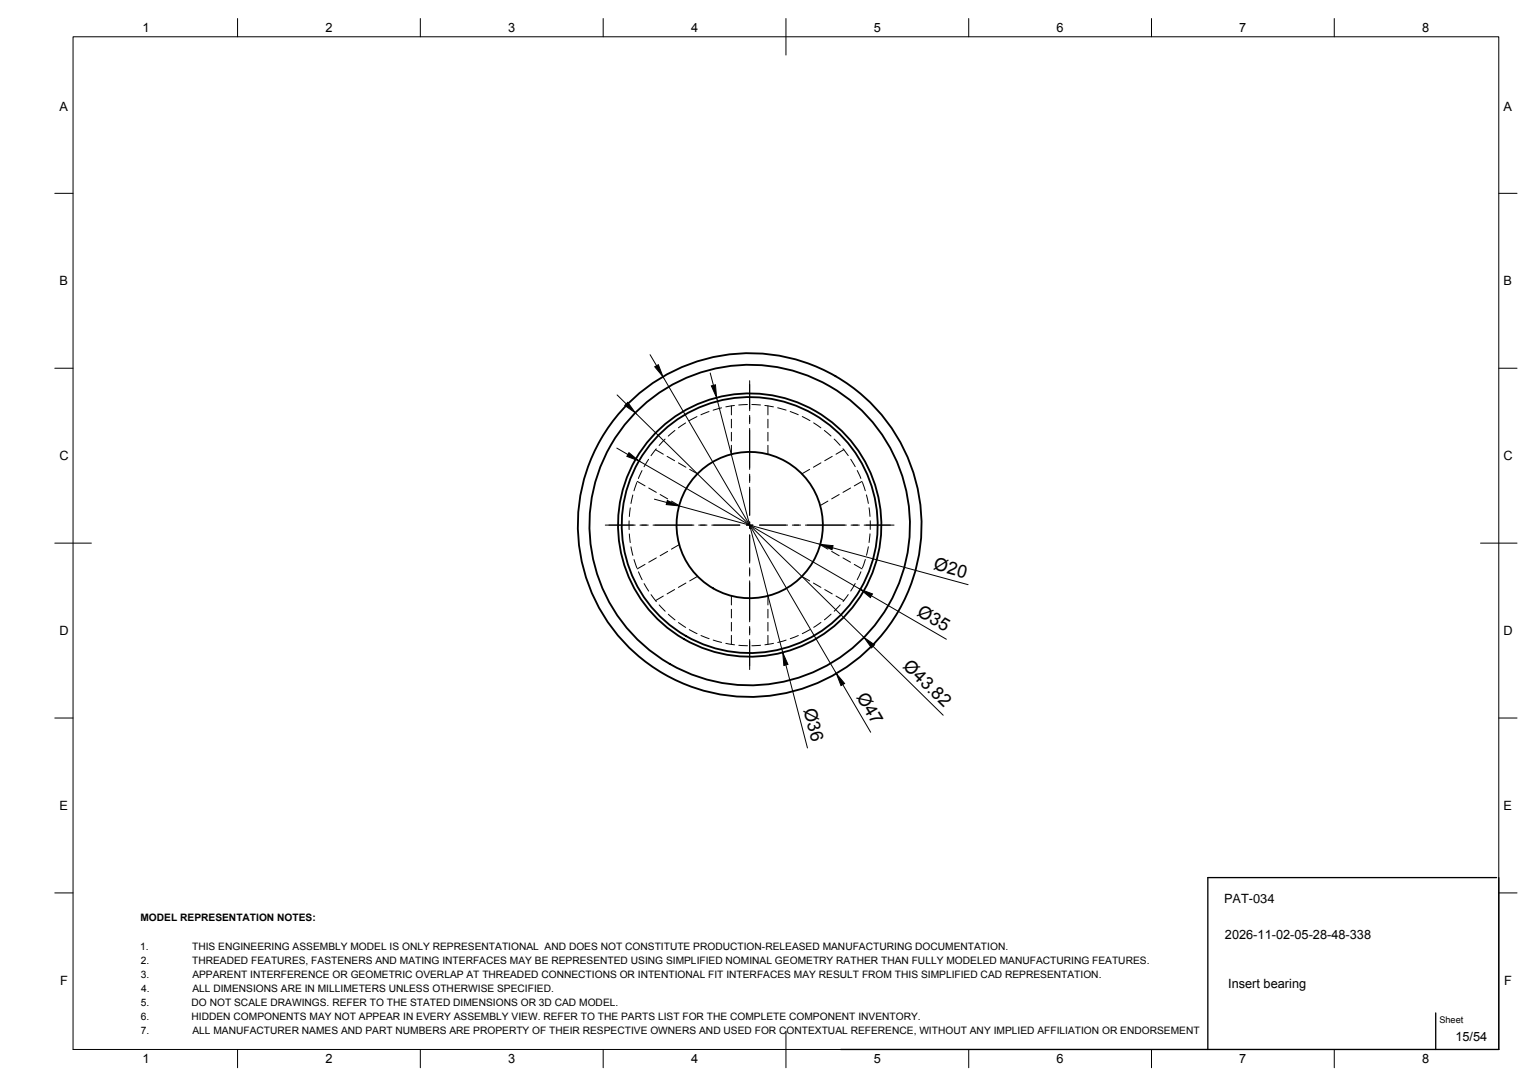
ISO-10303-21;
HEADER;
/* Generated by software containing ST-Developer
 * from STEP Tools, Inc. (www.steptools.com) 
 */

FILE_DESCRIPTION(
/* description */ ('Fatigue rig crank-slider'),
/* implementation_level */ '2;1');

FILE_NAME(
/* name */ 'Insert bearing.step',
/* time_stamp */ '2026-10-28T03:24:50-07:00',
/* author */ (''),
/* organization */ (''),
/* preprocessor_version */ 'ST-DEVELOPER v20.2',
/* originating_system */ 'Autodesk Translation Framework v15.17.0.0',
/* authorisation */ '');

FILE_SCHEMA (('AUTOMOTIVE_DESIGN { 1 0 10303 214 3 1 1 }'));
ENDSEC;

DATA;
#10=MECHANICAL_DESIGN_GEOMETRIC_PRESENTATION_REPRESENTATION('',(#598,#599),#16911);
#415=B_SPLINE_CURVE_WITH_KNOTS('',3,(#14016,#14017,#14018,#14019,#14020,
#14021,#14022,#14023,#14024,#14025),.UNSPECIFIED.,.F.,.F.,(4,2,2,2,4),(1.13193471301885,
1.22626174930539,1.32058878559194,1.41491753480854,1.50924628402513),
 .UNSPECIFIED.);
#416=B_SPLINE_CURVE_WITH_KNOTS('',3,(#14027,#14028,#14029,#14030,#14031,
#14032,#14033,#14034,#14035,#14036,#14037,#14038,#14039,#14040,#14041,#14042,
#14043,#14044),.UNSPECIFIED.,.F.,.F.,(4,2,2,2,2,2,2,2,4),(0.377311571006283,
0.471638607292829,0.565965643579376,0.66029439279597,0.754623142012565,
0.84895189122916,0.943280640445754,1.0376076767323,1.13193471301885),
 .UNSPECIFIED.);
#417=B_SPLINE_CURVE_WITH_KNOTS('',3,(#14045,#14046,#14047,#14048,#14049,
#14050,#14051,#14052,#14053,#14054),.UNSPECIFIED.,.F.,.F.,(4,2,2,2,4),(1.50924628402513,
1.60357503324173,1.69790378245832,1.79223081874487,1.88655785503141),
 .UNSPECIFIED.);
#418=B_SPLINE_CURVE_WITH_KNOTS('',3,(#14057,#14058,#14059,#14060,#14061,
#14062,#14063,#14064,#14065,#14066,#14067,#14068,#14069,#14070,#14071,#14072,
#14073,#14074,#14075,#14076,#14077,#14078,#14079,#14080,#14081,#14082,#14083,
#14084,#14085,#14086,#14087,#14088,#14089,#14090),.UNSPECIFIED.,.T.,.F.,
(4,2,2,2,2,2,2,2,2,2,2,2,2,2,2,2,4),(0.,0.0946120580087934,0.189224116017587,
0.283822945575014,0.378421775132442,0.47302060468987,0.567619434247297,
0.662231492256091,0.756843550264884,0.851455608273677,0.94606766628247,
1.0406664958399,1.13526532539733,1.22986415495475,1.32446298451218,1.41907504252097,
1.51368710052977),.UNSPECIFIED.);
#419=B_SPLINE_CURVE_WITH_KNOTS('',3,(#14093,#14094,#14095,#14096,#14097,
#14098,#14099,#14100,#14101,#14102,#14103,#14104,#14105,#14106,#14107,#14108,
#14109,#14110,#14111,#14112,#14113,#14114,#14115,#14116,#14117,#14118,#14119,
#14120,#14121,#14122,#14123,#14124,#14125,#14126),.UNSPECIFIED.,.T.,.F.,
(4,2,2,2,2,2,2,2,2,2,2,2,2,2,2,2,4),(0.,0.0946120580087934,0.189224116017587,
0.283822945575014,0.378421775132442,0.47302060468987,0.567619434247297,
0.66223149225609,0.756843550264884,0.851455608273677,0.94606766628247,1.0406664958399,
1.13526532539733,1.22986415495475,1.32446298451218,1.41907504252097,1.51368710052977),
 .UNSPECIFIED.);
#420=B_SPLINE_CURVE_WITH_KNOTS('',3,(#14130,#14131,#14132,#14133,#14134,
#14135,#14136,#14137,#14138,#14139),.UNSPECIFIED.,.F.,.F.,(4,2,2,2,4),(1.13193471301885,
1.22626174930539,1.32058878559194,1.41491753480854,1.50924628402513),
 .UNSPECIFIED.);
#421=B_SPLINE_CURVE_WITH_KNOTS('',3,(#14141,#14142,#14143,#14144,#14145,
#14146,#14147,#14148,#14149,#14150,#14151,#14152,#14153,#14154,#14155,#14156,
#14157,#14158),.UNSPECIFIED.,.F.,.F.,(4,2,2,2,2,2,2,2,4),(0.377311571006283,
0.47163860729283,0.565965643579376,0.660294392795971,0.754623142012565,
0.84895189122916,0.943280640445755,1.0376076767323,1.13193471301885),
 .UNSPECIFIED.);
#422=B_SPLINE_CURVE_WITH_KNOTS('',3,(#14159,#14160,#14161,#14162,#14163,
#14164,#14165,#14166,#14167,#14168),.UNSPECIFIED.,.F.,.F.,(4,2,2,2,4),(1.50924628402513,
1.60357503324173,1.69790378245832,1.79223081874487,1.88655785503141),
 .UNSPECIFIED.);
#423=B_SPLINE_CURVE_WITH_KNOTS('',3,(#14177,#14178,#14179,#14180,#14181,
#14182,#14183,#14184,#14185,#14186,#14187,#14188,#14189,#14190,#14191,#14192,
#14193,#14194),.UNSPECIFIED.,.F.,.F.,(4,2,2,2,2,2,2,2,4),(0.377311571006282,
0.471638607292829,0.565965643579376,0.660294392795971,0.754623142012565,
0.84895189122916,0.943280640445754,1.0376076767323,1.13193471301885),
 .UNSPECIFIED.);
#424=B_SPLINE_CURVE_WITH_KNOTS('',3,(#14196,#14197,#14198,#14199,#14200,
#14201,#14202,#14203,#14204,#14205),.UNSPECIFIED.,.F.,.F.,(4,2,2,2,4),(1.13193471301885,
1.22626174930539,1.32058878559194,1.41491753480854,1.50924628402513),
 .UNSPECIFIED.);
#425=B_SPLINE_CURVE_WITH_KNOTS('',3,(#14206,#14207,#14208,#14209,#14210,
#14211,#14212,#14213,#14214,#14215),.UNSPECIFIED.,.F.,.F.,(4,2,2,2,4),(1.50924628402513,
1.60357503324172,1.69790378245832,1.79223081874487,1.88655785503141),
 .UNSPECIFIED.);
#426=B_SPLINE_CURVE_WITH_KNOTS('',3,(#14218,#14219,#14220,#14221,#14222,
#14223,#14224,#14225,#14226,#14227,#14228,#14229,#14230,#14231,#14232,#14233,
#14234,#14235),.UNSPECIFIED.,.F.,.F.,(4,2,2,2,2,2,2,2,4),(0.377311571006283,
0.47163860729283,0.565965643579376,0.660294392795971,0.754623142012565,
0.84895189122916,0.943280640445754,1.0376076767323,1.13193471301885),
 .UNSPECIFIED.);
#427=B_SPLINE_CURVE_WITH_KNOTS('',3,(#14237,#14238,#14239,#14240,#14241,
#14242,#14243,#14244,#14245,#14246),.UNSPECIFIED.,.F.,.F.,(4,2,2,2,4),(1.13193471301885,
1.22626174930539,1.32058878559194,1.41491753480854,1.50924628402513),
 .UNSPECIFIED.);
#428=B_SPLINE_CURVE_WITH_KNOTS('',3,(#14247,#14248,#14249,#14250,#14251,
#14252,#14253,#14254,#14255,#14256),.UNSPECIFIED.,.F.,.F.,(4,2,2,2,4),(1.50924628402513,
1.60357503324173,1.69790378245832,1.79223081874487,1.88655785503141),
 .UNSPECIFIED.);
#429=B_SPLINE_CURVE_WITH_KNOTS('',3,(#14259,#14260,#14261,#14262,#14263,
#14264,#14265,#14266,#14267,#14268,#14269,#14270,#14271,#14272,#14273,#14274,
#14275,#14276),.UNSPECIFIED.,.F.,.F.,(4,2,2,2,2,2,2,2,4),(0.377311571006282,
0.471638607292829,0.565965643579376,0.66029439279597,0.754623142012565,
0.84895189122916,0.943280640445754,1.0376076767323,1.13193471301885),
 .UNSPECIFIED.);
#430=B_SPLINE_CURVE_WITH_KNOTS('',3,(#14278,#14279,#14280,#14281,#14282,
#14283,#14284,#14285,#14286,#14287),.UNSPECIFIED.,.F.,.F.,(4,2,2,2,4),(1.13193471301885,
1.22626174930539,1.32058878559194,1.41491753480854,1.50924628402513),
 .UNSPECIFIED.);
#431=B_SPLINE_CURVE_WITH_KNOTS('',3,(#14288,#14289,#14290,#14291,#14292,
#14293,#14294,#14295,#14296,#14297),.UNSPECIFIED.,.F.,.F.,(4,2,2,2,4),(1.50924628402513,
1.60357503324172,1.69790378245832,1.79223081874487,1.88655785503141),
 .UNSPECIFIED.);
#432=B_SPLINE_CURVE_WITH_KNOTS('',3,(#14300,#14301,#14302,#14303,#14304,
#14305,#14306,#14307,#14308,#14309,#14310,#14311,#14312,#14313,#14314,#14315,
#14316,#14317),.UNSPECIFIED.,.F.,.F.,(4,2,2,2,2,2,2,2,4),(0.377311571006283,
0.471638607292829,0.565965643579376,0.660294392795971,0.754623142012565,
0.84895189122916,0.943280640445755,1.0376076767323,1.13193471301885),
 .UNSPECIFIED.);
#433=B_SPLINE_CURVE_WITH_KNOTS('',3,(#14319,#14320,#14321,#14322,#14323,
#14324,#14325,#14326,#14327,#14328),.UNSPECIFIED.,.F.,.F.,(4,2,2,2,4),(1.13193471301885,
1.22626174930539,1.32058878559194,1.41491753480854,1.50924628402513),
 .UNSPECIFIED.);
#434=B_SPLINE_CURVE_WITH_KNOTS('',3,(#14329,#14330,#14331,#14332,#14333,
#14334,#14335,#14336,#14337,#14338),.UNSPECIFIED.,.F.,.F.,(4,2,2,2,4),(1.50924628402513,
1.60357503324172,1.69790378245832,1.79223081874487,1.88655785503141),
 .UNSPECIFIED.);
#435=B_SPLINE_CURVE_WITH_KNOTS('',3,(#14342,#14343,#14344,#14345,#14346,
#14347,#14348,#14349,#14350,#14351,#14352,#14353,#14354,#14355,#14356,#14357,
#14358,#14359,#14360,#14361,#14362,#14363,#14364,#14365,#14366,#14367,#14368,
#14369,#14370,#14371,#14372,#14373,#14374,#14375),.UNSPECIFIED.,.T.,.F.,
(4,2,2,2,2,2,2,2,2,2,2,2,2,2,2,2,4),(0.,0.0946120580087934,0.189224116017587,
0.283822945575014,0.378421775132442,0.47302060468987,0.567619434247297,
0.66223149225609,0.756843550264884,0.851455608273677,0.94606766628247,1.0406664958399,
1.13526532539733,1.22986415495475,1.32446298451218,1.41907504252097,1.51368710052977),
 .UNSPECIFIED.);
#436=B_SPLINE_CURVE_WITH_KNOTS('',3,(#14378,#14379,#14380,#14381,#14382,
#14383,#14384,#14385,#14386,#14387,#14388,#14389,#14390,#14391,#14392,#14393,
#14394,#14395,#14396,#14397,#14398,#14399,#14400,#14401,#14402,#14403,#14404,
#14405,#14406,#14407,#14408,#14409,#14410,#14411),.UNSPECIFIED.,.T.,.F.,
(4,2,2,2,2,2,2,2,2,2,2,2,2,2,2,2,4),(0.,0.0946120580087934,0.189224116017587,
0.283822945575014,0.378421775132442,0.47302060468987,0.567619434247297,
0.66223149225609,0.756843550264884,0.851455608273677,0.94606766628247,1.0406664958399,
1.13526532539733,1.22986415495475,1.32446298451218,1.41907504252097,1.51368710052977),
 .UNSPECIFIED.);
#437=B_SPLINE_CURVE_WITH_KNOTS('',3,(#14416,#14417,#14418,#14419,#14420,
#14421,#14422,#14423,#14424,#14425,#14426,#14427,#14428,#14429,#14430,#14431,
#14432,#14433,#14434,#14435,#14436,#14437,#14438,#14439,#14440,#14441,#14442,
#14443,#14444,#14445,#14446,#14447,#14448,#14449),.UNSPECIFIED.,.T.,.F.,
(4,2,2,2,2,2,2,2,2,2,2,2,2,2,2,2,4),(0.,0.0946120580087934,0.189224116017587,
0.283822945575014,0.378421775132442,0.47302060468987,0.567619434247297,
0.66223149225609,0.756843550264884,0.851455608273677,0.94606766628247,1.0406664958399,
1.13526532539733,1.22986415495475,1.32446298451218,1.41907504252097,1.51368710052977),
 .UNSPECIFIED.);
#438=B_SPLINE_CURVE_WITH_KNOTS('',3,(#14452,#14453,#14454,#14455,#14456,
#14457,#14458,#14459,#14460,#14461,#14462,#14463,#14464,#14465,#14466,#14467,
#14468,#14469,#14470,#14471,#14472,#14473,#14474,#14475,#14476,#14477,#14478,
#14479,#14480,#14481,#14482,#14483,#14484,#14485),.UNSPECIFIED.,.T.,.F.,
(4,2,2,2,2,2,2,2,2,2,2,2,2,2,2,2,4),(0.,0.0946120580087934,0.189224116017587,
0.283822945575014,0.378421775132442,0.47302060468987,0.567619434247297,
0.66223149225609,0.756843550264884,0.851455608273677,0.94606766628247,1.0406664958399,
1.13526532539733,1.22986415495475,1.32446298451218,1.41907504252097,1.51368710052977),
 .UNSPECIFIED.);
#470=SPHERICAL_SURFACE('',#9773,2.35);
#498=SHAPE_REPRESENTATION_RELATIONSHIP('SRR','None',#17138,#548);
#548=ADVANCED_BREP_SHAPE_REPRESENTATION('',(#657,#658),#16867);
#598=STYLED_ITEM('',(#17487),#657);
#599=STYLED_ITEM('',(#17487),#658);
#657=MANIFOLD_SOLID_BREP('Body1',#8889);
#658=MANIFOLD_SOLID_BREP('Body2',#8890);
#786=FACE_BOUND('',#1969,.T.);
#787=FACE_BOUND('',#1971,.T.);
#788=FACE_BOUND('',#1972,.T.);
#789=FACE_BOUND('',#1974,.T.);
#790=FACE_BOUND('',#1978,.T.);
#791=FACE_BOUND('',#1979,.T.);
#792=FACE_BOUND('',#1980,.T.);
#793=FACE_BOUND('',#1981,.T.);
#794=FACE_BOUND('',#1982,.T.);
#795=FACE_BOUND('',#1983,.T.);
#796=FACE_BOUND('',#1989,.T.);
#797=FACE_BOUND('',#1991,.T.);
#798=FACE_BOUND('',#1994,.T.);
#799=FACE_BOUND('',#1996,.T.);
#800=FACE_BOUND('',#1997,.T.);
#801=FACE_BOUND('',#1998,.T.);
#802=FACE_BOUND('',#1999,.T.);
#803=FACE_BOUND('',#2000,.T.);
#804=FACE_BOUND('',#2001,.T.);
#980=PLANE('',#9771);
#981=PLANE('',#9776);
#982=PLANE('',#9786);
#983=PLANE('',#9788);
#984=PLANE('',#9792);
#1358=FACE_OUTER_BOUND('',#1967,.T.);
#1359=FACE_OUTER_BOUND('',#1968,.T.);
#1360=FACE_OUTER_BOUND('',#1970,.T.);
#1361=FACE_OUTER_BOUND('',#1973,.T.);
#1362=FACE_OUTER_BOUND('',#1975,.T.);
#1363=FACE_OUTER_BOUND('',#1976,.T.);
#1364=FACE_OUTER_BOUND('',#1977,.T.);
#1365=FACE_OUTER_BOUND('',#1984,.T.);
#1366=FACE_OUTER_BOUND('',#1985,.T.);
#1367=FACE_OUTER_BOUND('',#1986,.T.);
#1368=FACE_OUTER_BOUND('',#1987,.T.);
#1369=FACE_OUTER_BOUND('',#1988,.T.);
#1370=FACE_OUTER_BOUND('',#1990,.T.);
#1371=FACE_OUTER_BOUND('',#1992,.T.);
#1372=FACE_OUTER_BOUND('',#1993,.T.);
#1373=FACE_OUTER_BOUND('',#1995,.T.);
#1967=EDGE_LOOP('',(#6574,#6575,#6576,#6577));
#1968=EDGE_LOOP('',(#6578));
#1969=EDGE_LOOP('',(#6579));
#1970=EDGE_LOOP('',(#6580,#6581));
#1971=EDGE_LOOP('',(#6582));
#1972=EDGE_LOOP('',(#6583));
#1973=EDGE_LOOP('',(#6584));
#1974=EDGE_LOOP('',(#6585));
#1975=EDGE_LOOP('',(#6586,#6587,#6588,#6589,#6590,#6591));
#1976=EDGE_LOOP('',(#6592,#6593,#6594,#6595,#6596,#6597));
#1977=EDGE_LOOP('',(#6598,#6599,#6600,#6601));
#1978=EDGE_LOOP('',(#6602,#6603,#6604));
#1979=EDGE_LOOP('',(#6605,#6606,#6607));
#1980=EDGE_LOOP('',(#6608,#6609,#6610));
#1981=EDGE_LOOP('',(#6611,#6612,#6613));
#1982=EDGE_LOOP('',(#6614,#6615,#6616));
#1983=EDGE_LOOP('',(#6617,#6618,#6619));
#1984=EDGE_LOOP('',(#6620,#6621,#6622,#6623,#6624,#6625));
#1985=EDGE_LOOP('',(#6626,#6627,#6628,#6629,#6630,#6631));
#1986=EDGE_LOOP('',(#6632,#6633,#6634,#6635,#6636,#6637));
#1987=EDGE_LOOP('',(#6638,#6639,#6640,#6641,#6642,#6643));
#1988=EDGE_LOOP('',(#6644));
#1989=EDGE_LOOP('',(#6645));
#1990=EDGE_LOOP('',(#6646));
#1991=EDGE_LOOP('',(#6647));
#1992=EDGE_LOOP('',(#6648,#6649,#6650,#6651));
#1993=EDGE_LOOP('',(#6652));
#1994=EDGE_LOOP('',(#6653));
#1995=EDGE_LOOP('',(#6654,#6655,#6656,#6657));
#1996=EDGE_LOOP('',(#6658));
#1997=EDGE_LOOP('',(#6659));
#1998=EDGE_LOOP('',(#6660));
#1999=EDGE_LOOP('',(#6661));
#2000=EDGE_LOOP('',(#6662));
#2001=EDGE_LOOP('',(#6663));
#2630=LINE('',#14001,#3276);
#2631=LINE('',#14056,#3277);
#2632=LINE('',#14128,#3278);
#2633=LINE('',#14173,#3279);
#2634=LINE('',#14341,#3280);
#2635=LINE('',#14412,#3281);
#2636=LINE('',#14415,#3282);
#2637=LINE('',#14486,#3283);
#2638=LINE('',#14496,#3284);
#2639=LINE('',#14501,#3285);
#3276=VECTOR('',#11290,1.8);
#3277=VECTOR('',#11307,0.25);
#3278=VECTOR('',#11310,0.25);
#3279=VECTOR('',#11315,1.65);
#3280=VECTOR('',#11320,0.25);
#3281=VECTOR('',#11323,0.25);
#3282=VECTOR('',#11326,0.25);
#3283=VECTOR('',#11329,0.25);
#3284=VECTOR('',#11342,1.75);
#3285=VECTOR('',#11349,1.);
#3871=CIRCLE('',#9769,1.8);
#3872=CIRCLE('',#9770,1.8);
#3873=CIRCLE('',#9772,2.19089023002066);
#3874=CIRCLE('',#9774,2.35);
#3875=CIRCLE('',#9775,2.19089023002066);
#3876=CIRCLE('',#9780,1.65);
#3877=CIRCLE('',#9781,1.65);
#3878=CIRCLE('',#9787,1.);
#3879=CIRCLE('',#9789,1.75);
#3880=CIRCLE('',#9791,1.75);
#3881=CIRCLE('',#9793,1.);
#4346=VERTEX_POINT('',#13998);
#4347=VERTEX_POINT('',#14000);
#4348=VERTEX_POINT('',#14004);
#4349=VERTEX_POINT('',#14007);
#4350=VERTEX_POINT('',#14008);
#4351=VERTEX_POINT('',#14010);
#4352=VERTEX_POINT('',#14014);
#4353=VERTEX_POINT('',#14015);
#4354=VERTEX_POINT('',#14026);
#4355=VERTEX_POINT('',#14055);
#4356=VERTEX_POINT('',#14092);
#4357=VERTEX_POINT('',#14127);
#4358=VERTEX_POINT('',#14129);
#4359=VERTEX_POINT('',#14140);
#4360=VERTEX_POINT('',#14170);
#4361=VERTEX_POINT('',#14172);
#4362=VERTEX_POINT('',#14175);
#4363=VERTEX_POINT('',#14176);
#4364=VERTEX_POINT('',#14195);
#4365=VERTEX_POINT('',#14216);
#4366=VERTEX_POINT('',#14217);
#4367=VERTEX_POINT('',#14236);
#4368=VERTEX_POINT('',#14257);
#4369=VERTEX_POINT('',#14258);
#4370=VERTEX_POINT('',#14277);
#4371=VERTEX_POINT('',#14298);
#4372=VERTEX_POINT('',#14299);
#4373=VERTEX_POINT('',#14318);
#4374=VERTEX_POINT('',#14340);
#4375=VERTEX_POINT('',#14377);
#4376=VERTEX_POINT('',#14414);
#4377=VERTEX_POINT('',#14451);
#4378=VERTEX_POINT('',#14488);
#4379=VERTEX_POINT('',#14491);
#4380=VERTEX_POINT('',#14494);
#4381=VERTEX_POINT('',#14498);
#5185=EDGE_CURVE('',#4346,#4346,#3871,.T.);
#5186=EDGE_CURVE('',#4346,#4347,#2630,.T.);
#5187=EDGE_CURVE('',#4347,#4347,#3872,.T.);
#5188=EDGE_CURVE('',#4348,#4348,#3873,.T.);
#5189=EDGE_CURVE('',#4349,#4350,#3874,.T.);
#5190=EDGE_CURVE('',#4351,#4351,#3875,.T.);
#5191=EDGE_CURVE('',#4352,#4353,#415,.T.);
#5192=EDGE_CURVE('',#4354,#4352,#416,.T.);
#5193=EDGE_CURVE('',#4353,#4354,#417,.T.);
#5194=EDGE_CURVE('',#4353,#4355,#2631,.T.);
#5195=EDGE_CURVE('',#4355,#4355,#418,.T.);
#5196=EDGE_CURVE('',#4356,#4356,#419,.T.);
#5197=EDGE_CURVE('',#4356,#4357,#2632,.T.);
#5198=EDGE_CURVE('',#4358,#4357,#420,.T.);
#5199=EDGE_CURVE('',#4359,#4358,#421,.T.);
#5200=EDGE_CURVE('',#4357,#4359,#422,.T.);
#5201=EDGE_CURVE('',#4360,#4360,#3876,.T.);
#5202=EDGE_CURVE('',#4360,#4361,#2633,.T.);
#5203=EDGE_CURVE('',#4361,#4361,#3877,.T.);
#5204=EDGE_CURVE('',#4362,#4363,#423,.T.);
#5205=EDGE_CURVE('',#4363,#4364,#424,.T.);
#5206=EDGE_CURVE('',#4364,#4362,#425,.T.);
#5207=EDGE_CURVE('',#4365,#4366,#426,.T.);
#5208=EDGE_CURVE('',#4366,#4367,#427,.T.);
#5209=EDGE_CURVE('',#4367,#4365,#428,.T.);
#5210=EDGE_CURVE('',#4368,#4369,#429,.T.);
#5211=EDGE_CURVE('',#4369,#4370,#430,.T.);
#5212=EDGE_CURVE('',#4370,#4368,#431,.T.);
#5213=EDGE_CURVE('',#4371,#4372,#432,.T.);
#5214=EDGE_CURVE('',#4372,#4373,#433,.T.);
#5215=EDGE_CURVE('',#4373,#4371,#434,.T.);
#5216=EDGE_CURVE('',#4364,#4374,#2634,.T.);
#5217=EDGE_CURVE('',#4374,#4374,#435,.T.);
#5218=EDGE_CURVE('',#4375,#4375,#436,.T.);
#5219=EDGE_CURVE('',#4375,#4367,#2635,.T.);
#5220=EDGE_CURVE('',#4370,#4376,#2636,.T.);
#5221=EDGE_CURVE('',#4376,#4376,#437,.T.);
#5222=EDGE_CURVE('',#4377,#4377,#438,.T.);
#5223=EDGE_CURVE('',#4377,#4373,#2637,.T.);
#5224=EDGE_CURVE('',#4378,#4378,#3878,.T.);
#5225=EDGE_CURVE('',#4379,#4379,#3879,.T.);
#5226=EDGE_CURVE('',#4380,#4380,#3880,.T.);
#5227=EDGE_CURVE('',#4380,#4379,#2638,.T.);
#5228=EDGE_CURVE('',#4381,#4381,#3881,.T.);
#5229=EDGE_CURVE('',#4381,#4378,#2639,.T.);
#6574=ORIENTED_EDGE('',*,*,#5185,.T.);
#6575=ORIENTED_EDGE('',*,*,#5186,.T.);
#6576=ORIENTED_EDGE('',*,*,#5187,.F.);
#6577=ORIENTED_EDGE('',*,*,#5186,.F.);
#6578=ORIENTED_EDGE('',*,*,#5188,.F.);
#6579=ORIENTED_EDGE('',*,*,#5187,.T.);
#6580=ORIENTED_EDGE('',*,*,#5189,.T.);
#6581=ORIENTED_EDGE('',*,*,#5189,.F.);
#6582=ORIENTED_EDGE('',*,*,#5188,.T.);
#6583=ORIENTED_EDGE('',*,*,#5190,.F.);
#6584=ORIENTED_EDGE('',*,*,#5190,.T.);
#6585=ORIENTED_EDGE('',*,*,#5185,.F.);
#6586=ORIENTED_EDGE('',*,*,#5191,.F.);
#6587=ORIENTED_EDGE('',*,*,#5192,.F.);
#6588=ORIENTED_EDGE('',*,*,#5193,.F.);
#6589=ORIENTED_EDGE('',*,*,#5194,.T.);
#6590=ORIENTED_EDGE('',*,*,#5195,.F.);
#6591=ORIENTED_EDGE('',*,*,#5194,.F.);
#6592=ORIENTED_EDGE('',*,*,#5196,.F.);
#6593=ORIENTED_EDGE('',*,*,#5197,.T.);
#6594=ORIENTED_EDGE('',*,*,#5198,.F.);
#6595=ORIENTED_EDGE('',*,*,#5199,.F.);
#6596=ORIENTED_EDGE('',*,*,#5200,.F.);
#6597=ORIENTED_EDGE('',*,*,#5197,.F.);
#6598=ORIENTED_EDGE('',*,*,#5201,.F.);
#6599=ORIENTED_EDGE('',*,*,#5202,.T.);
#6600=ORIENTED_EDGE('',*,*,#5203,.T.);
#6601=ORIENTED_EDGE('',*,*,#5202,.F.);
#6602=ORIENTED_EDGE('',*,*,#5192,.T.);
#6603=ORIENTED_EDGE('',*,*,#5191,.T.);
#6604=ORIENTED_EDGE('',*,*,#5193,.T.);
#6605=ORIENTED_EDGE('',*,*,#5199,.T.);
#6606=ORIENTED_EDGE('',*,*,#5198,.T.);
#6607=ORIENTED_EDGE('',*,*,#5200,.T.);
#6608=ORIENTED_EDGE('',*,*,#5204,.T.);
#6609=ORIENTED_EDGE('',*,*,#5205,.T.);
#6610=ORIENTED_EDGE('',*,*,#5206,.T.);
#6611=ORIENTED_EDGE('',*,*,#5207,.T.);
#6612=ORIENTED_EDGE('',*,*,#5208,.T.);
#6613=ORIENTED_EDGE('',*,*,#5209,.T.);
#6614=ORIENTED_EDGE('',*,*,#5210,.T.);
#6615=ORIENTED_EDGE('',*,*,#5211,.T.);
#6616=ORIENTED_EDGE('',*,*,#5212,.T.);
#6617=ORIENTED_EDGE('',*,*,#5213,.T.);
#6618=ORIENTED_EDGE('',*,*,#5214,.T.);
#6619=ORIENTED_EDGE('',*,*,#5215,.T.);
#6620=ORIENTED_EDGE('',*,*,#5205,.F.);
#6621=ORIENTED_EDGE('',*,*,#5204,.F.);
#6622=ORIENTED_EDGE('',*,*,#5206,.F.);
#6623=ORIENTED_EDGE('',*,*,#5216,.T.);
#6624=ORIENTED_EDGE('',*,*,#5217,.F.);
#6625=ORIENTED_EDGE('',*,*,#5216,.F.);
#6626=ORIENTED_EDGE('',*,*,#5218,.F.);
#6627=ORIENTED_EDGE('',*,*,#5219,.T.);
#6628=ORIENTED_EDGE('',*,*,#5208,.F.);
#6629=ORIENTED_EDGE('',*,*,#5207,.F.);
#6630=ORIENTED_EDGE('',*,*,#5209,.F.);
#6631=ORIENTED_EDGE('',*,*,#5219,.F.);
#6632=ORIENTED_EDGE('',*,*,#5211,.F.);
#6633=ORIENTED_EDGE('',*,*,#5210,.F.);
#6634=ORIENTED_EDGE('',*,*,#5212,.F.);
#6635=ORIENTED_EDGE('',*,*,#5220,.T.);
#6636=ORIENTED_EDGE('',*,*,#5221,.F.);
#6637=ORIENTED_EDGE('',*,*,#5220,.F.);
#6638=ORIENTED_EDGE('',*,*,#5222,.F.);
#6639=ORIENTED_EDGE('',*,*,#5223,.T.);
#6640=ORIENTED_EDGE('',*,*,#5214,.F.);
#6641=ORIENTED_EDGE('',*,*,#5213,.F.);
#6642=ORIENTED_EDGE('',*,*,#5215,.F.);
#6643=ORIENTED_EDGE('',*,*,#5223,.F.);
#6644=ORIENTED_EDGE('',*,*,#5203,.F.);
#6645=ORIENTED_EDGE('',*,*,#5224,.T.);
#6646=ORIENTED_EDGE('',*,*,#5225,.F.);
#6647=ORIENTED_EDGE('',*,*,#5201,.T.);
#6648=ORIENTED_EDGE('',*,*,#5226,.F.);
#6649=ORIENTED_EDGE('',*,*,#5227,.T.);
#6650=ORIENTED_EDGE('',*,*,#5225,.T.);
#6651=ORIENTED_EDGE('',*,*,#5227,.F.);
#6652=ORIENTED_EDGE('',*,*,#5226,.T.);
#6653=ORIENTED_EDGE('',*,*,#5228,.F.);
#6654=ORIENTED_EDGE('',*,*,#5228,.T.);
#6655=ORIENTED_EDGE('',*,*,#5229,.T.);
#6656=ORIENTED_EDGE('',*,*,#5224,.F.);
#6657=ORIENTED_EDGE('',*,*,#5229,.F.);
#6658=ORIENTED_EDGE('',*,*,#5196,.T.);
#6659=ORIENTED_EDGE('',*,*,#5195,.T.);
#6660=ORIENTED_EDGE('',*,*,#5218,.T.);
#6661=ORIENTED_EDGE('',*,*,#5217,.T.);
#6662=ORIENTED_EDGE('',*,*,#5222,.T.);
#6663=ORIENTED_EDGE('',*,*,#5221,.T.);
#8253=CYLINDRICAL_SURFACE('',#9768,1.8);
#8254=CYLINDRICAL_SURFACE('',#9777,0.25);
#8255=CYLINDRICAL_SURFACE('',#9778,0.25);
#8256=CYLINDRICAL_SURFACE('',#9779,1.65);
#8257=CYLINDRICAL_SURFACE('',#9782,0.25);
#8258=CYLINDRICAL_SURFACE('',#9783,0.25);
#8259=CYLINDRICAL_SURFACE('',#9784,0.25);
#8260=CYLINDRICAL_SURFACE('',#9785,0.25);
#8261=CYLINDRICAL_SURFACE('',#9790,1.75);
#8262=CYLINDRICAL_SURFACE('',#9794,1.);
#8496=ADVANCED_FACE('',(#1358),#8253,.F.);
#8497=ADVANCED_FACE('',(#1359,#786),#980,.T.);
#8498=ADVANCED_FACE('',(#1360,#787,#788),#470,.T.);
#8499=ADVANCED_FACE('',(#1361,#789),#981,.T.);
#8500=ADVANCED_FACE('',(#1362),#8254,.F.);
#8501=ADVANCED_FACE('',(#1363),#8255,.F.);
#8502=ADVANCED_FACE('',(#1364,#790,#791,#792,#793,#794,#795),#8256,.T.);
#8503=ADVANCED_FACE('',(#1365),#8257,.F.);
#8504=ADVANCED_FACE('',(#1366),#8258,.F.);
#8505=ADVANCED_FACE('',(#1367),#8259,.F.);
#8506=ADVANCED_FACE('',(#1368),#8260,.F.);
#8507=ADVANCED_FACE('',(#1369,#796),#982,.T.);
#8508=ADVANCED_FACE('',(#1370,#797),#983,.T.);
#8509=ADVANCED_FACE('',(#1371),#8261,.T.);
#8510=ADVANCED_FACE('',(#1372,#798),#984,.T.);
#8511=ADVANCED_FACE('',(#1373,#799,#800,#801,#802,#803,#804),#8262,.F.);
#8889=CLOSED_SHELL('',(#8496,#8497,#8498,#8499));
#8890=CLOSED_SHELL('',(#8500,#8501,#8502,#8503,#8504,#8505,#8506,#8507,
#8508,#8509,#8510,#8511));
#9767=AXIS2_PLACEMENT_3D('',#13996,#11284,#11285);
#9768=AXIS2_PLACEMENT_3D('',#13997,#11286,#11287);
#9769=AXIS2_PLACEMENT_3D('',#13999,#11288,#11289);
#9770=AXIS2_PLACEMENT_3D('',#14002,#11291,#11292);
#9771=AXIS2_PLACEMENT_3D('',#14003,#11293,#11294);
#9772=AXIS2_PLACEMENT_3D('',#14005,#11295,#11296);
#9773=AXIS2_PLACEMENT_3D('',#14006,#11297,#11298);
#9774=AXIS2_PLACEMENT_3D('',#14009,#11299,#11300);
#9775=AXIS2_PLACEMENT_3D('',#14011,#11301,#11302);
#9776=AXIS2_PLACEMENT_3D('',#14012,#11303,#11304);
#9777=AXIS2_PLACEMENT_3D('',#14013,#11305,#11306);
#9778=AXIS2_PLACEMENT_3D('',#14091,#11308,#11309);
#9779=AXIS2_PLACEMENT_3D('',#14169,#11311,#11312);
#9780=AXIS2_PLACEMENT_3D('',#14171,#11313,#11314);
#9781=AXIS2_PLACEMENT_3D('',#14174,#11316,#11317);
#9782=AXIS2_PLACEMENT_3D('',#14339,#11318,#11319);
#9783=AXIS2_PLACEMENT_3D('',#14376,#11321,#11322);
#9784=AXIS2_PLACEMENT_3D('',#14413,#11324,#11325);
#9785=AXIS2_PLACEMENT_3D('',#14450,#11327,#11328);
#9786=AXIS2_PLACEMENT_3D('',#14487,#11330,#11331);
#9787=AXIS2_PLACEMENT_3D('',#14489,#11332,#11333);
#9788=AXIS2_PLACEMENT_3D('',#14490,#11334,#11335);
#9789=AXIS2_PLACEMENT_3D('',#14492,#11336,#11337);
#9790=AXIS2_PLACEMENT_3D('',#14493,#11338,#11339);
#9791=AXIS2_PLACEMENT_3D('',#14495,#11340,#11341);
#9792=AXIS2_PLACEMENT_3D('',#14497,#11343,#11344);
#9793=AXIS2_PLACEMENT_3D('',#14499,#11345,#11346);
#9794=AXIS2_PLACEMENT_3D('',#14500,#11347,#11348);
#11284=DIRECTION('axis',(0.,0.,1.));
#11285=DIRECTION('refdir',(1.,0.,0.));
#11286=DIRECTION('center_axis',(0.,-1.,0.));
#11287=DIRECTION('ref_axis',(1.,0.,0.));
#11288=DIRECTION('center_axis',(0.,-1.,0.));
#11289=DIRECTION('ref_axis',(1.,0.,0.));
#11290=DIRECTION('',(0.,1.,0.));
#11291=DIRECTION('center_axis',(0.,-1.,0.));
#11292=DIRECTION('ref_axis',(1.,0.,0.));
#11293=DIRECTION('center_axis',(0.,1.,0.));
#11294=DIRECTION('ref_axis',(0.,0.,1.));
#11295=DIRECTION('center_axis',(0.,-1.,0.));
#11296=DIRECTION('ref_axis',(1.,0.,0.));
#11297=DIRECTION('center_axis',(6.12323399573677E-17,0.,1.));
#11298=DIRECTION('ref_axis',(1.,0.,0.));
#11299=DIRECTION('center_axis',(1.22464679914735E-16,-1.,0.));
#11300=DIRECTION('ref_axis',(-1.,-1.22464679914735E-16,0.));
#11301=DIRECTION('center_axis',(0.,-1.,0.));
#11302=DIRECTION('ref_axis',(1.,0.,0.));
#11303=DIRECTION('center_axis',(0.,-1.,0.));
#11304=DIRECTION('ref_axis',(0.,0.,-1.));
#11305=DIRECTION('center_axis',(-0.866025403784438,0.,-0.5));
#11306=DIRECTION('ref_axis',(-0.5,0.,0.866025403784438));
#11307=DIRECTION('',(-0.866025403784438,0.,-0.5));
#11308=DIRECTION('center_axis',(-0.866025403784438,0.,-0.5));
#11309=DIRECTION('ref_axis',(-0.5,0.,0.866025403784438));
#11310=DIRECTION('',(-0.866025403784438,0.,-0.5));
#11311=DIRECTION('center_axis',(0.,-1.,0.));
#11312=DIRECTION('ref_axis',(1.,0.,0.));
#11313=DIRECTION('center_axis',(0.,-1.,0.));
#11314=DIRECTION('ref_axis',(1.,0.,0.));
#11315=DIRECTION('',(0.,1.,0.));
#11316=DIRECTION('center_axis',(0.,-1.,0.));
#11317=DIRECTION('ref_axis',(1.,0.,0.));
#11318=DIRECTION('center_axis',(0.866025403784439,0.,-0.5));
#11319=DIRECTION('ref_axis',(-0.5,0.,-0.866025403784439));
#11320=DIRECTION('',(0.866025403784439,0.,-0.5));
#11321=DIRECTION('center_axis',(0.866025403784439,0.,-0.5));
#11322=DIRECTION('ref_axis',(-0.5,0.,-0.866025403784439));
#11323=DIRECTION('',(0.866025403784439,0.,-0.5));
#11324=DIRECTION('center_axis',(0.,0.,1.));
#11325=DIRECTION('ref_axis',(1.,0.,0.));
#11326=DIRECTION('',(0.,0.,1.));
#11327=DIRECTION('center_axis',(0.,0.,1.));
#11328=DIRECTION('ref_axis',(1.,0.,0.));
#11329=DIRECTION('',(0.,0.,1.));
#11330=DIRECTION('center_axis',(0.,1.,0.));
#11331=DIRECTION('ref_axis',(0.,0.,1.));
#11332=DIRECTION('center_axis',(0.,-1.,0.));
#11333=DIRECTION('ref_axis',(1.,0.,0.));
#11334=DIRECTION('center_axis',(0.,1.,0.));
#11335=DIRECTION('ref_axis',(0.,0.,1.));
#11336=DIRECTION('center_axis',(0.,-1.,0.));
#11337=DIRECTION('ref_axis',(1.,0.,0.));
#11338=DIRECTION('center_axis',(0.,-1.,0.));
#11339=DIRECTION('ref_axis',(1.,0.,0.));
#11340=DIRECTION('center_axis',(0.,-1.,0.));
#11341=DIRECTION('ref_axis',(1.,0.,0.));
#11342=DIRECTION('',(0.,1.,0.));
#11343=DIRECTION('center_axis',(0.,-1.,0.));
#11344=DIRECTION('ref_axis',(0.,0.,-1.));
#11345=DIRECTION('center_axis',(0.,-1.,0.));
#11346=DIRECTION('ref_axis',(1.,0.,0.));
#11347=DIRECTION('center_axis',(0.,-1.,0.));
#11348=DIRECTION('ref_axis',(1.,0.,0.));
#11349=DIRECTION('',(0.,1.,0.));
#13996=CARTESIAN_POINT('',(0.,0.,0.));
#13997=CARTESIAN_POINT('Origin',(0.,0.,0.));
#13998=CARTESIAN_POINT('',(-1.8,-0.85,-2.20436423846524E-16));
#13999=CARTESIAN_POINT('Origin',(0.,-0.85,0.));
#14000=CARTESIAN_POINT('',(-1.8,0.85,-2.20436423846524E-16));
#14001=CARTESIAN_POINT('',(-1.8,0.,-2.20436423846524E-16));
#14002=CARTESIAN_POINT('Origin',(0.,0.85,0.));
#14003=CARTESIAN_POINT('Origin',(2.19089023002066,0.85,0.));
#14004=CARTESIAN_POINT('',(2.19089023002066,0.85,0.));
#14005=CARTESIAN_POINT('Origin',(0.,0.85,0.));
#14006=CARTESIAN_POINT('Origin',(3.99680288865056E-15,0.,0.));
#14007=CARTESIAN_POINT('',(3.85290688975075E-15,-1.76221774462768E-32,2.35));
#14008=CARTESIAN_POINT('',(3.85290688975075E-15,-1.76221774462768E-32,-2.35));
#14009=CARTESIAN_POINT('Origin',(3.99680288865056E-15,0.,0.));
#14010=CARTESIAN_POINT('',(2.19089023002066,-0.85,0.));
#14011=CARTESIAN_POINT('Origin',(0.,-0.85,0.));
#14012=CARTESIAN_POINT('Origin',(1.8,-0.85,0.));
#14013=CARTESIAN_POINT('Origin',(0.,1.55,0.));
#14014=CARTESIAN_POINT('',(1.42894191624432,1.8,0.825000000000001));
#14015=CARTESIAN_POINT('',(1.53744468918255,1.55,0.598968970568896));
#14016=CARTESIAN_POINT('Ctrl Pts',(1.42894191624432,1.8,0.825000000000001));
#14017=CARTESIAN_POINT('Ctrl Pts',(1.44466308895875,1.8,0.797770130104052));
#14018=CARTESIAN_POINT('Ctrl Pts',(1.46055812562105,1.79370633789704,0.768258557763732));
#14019=CARTESIAN_POINT('Ctrl Pts',(1.48824888379079,1.76817777258318,0.713138492740816));
#14020=CARTESIAN_POINT('Ctrl Pts',(1.50008999307766,1.74894552961493,0.687551581002689));
#14021=CARTESIAN_POINT('Ctrl Pts',(1.51812136280714,1.70460745840382,0.646764802471699));
#14022=CARTESIAN_POINT('Ctrl Pts',(1.52552758004446,1.67652816181843,0.628833667319578));
#14023=CARTESIAN_POINT('Ctrl Pts',(1.53516661651472,1.61494799959182,0.604921184808251));
#14024=CARTESIAN_POINT('Ctrl Pts',(1.53744468918255,1.58144291640553,0.598968970568896));
#14025=CARTESIAN_POINT('Ctrl Pts',(1.53744468918255,1.55,0.598968970568896));
#14026=CARTESIAN_POINT('',(1.42894191624432,1.3,0.825000000000001));
#14027=CARTESIAN_POINT('Ctrl Pts',(1.42894191624432,1.3,0.825000000000001));
#14028=CARTESIAN_POINT('Ctrl Pts',(1.4132207435299,1.3,0.852229869895949));
#14029=CARTESIAN_POINT('Ctrl Pts',(1.39561049050871,1.30629366210296,0.880751161609749));
#14030=CARTESIAN_POINT('Ctrl Pts',(1.36172049302549,1.33182222741682,0.932292094146256));
#14031=CARTESIAN_POINT('Ctrl Pts',(1.34548213209931,1.35105447038507,0.955340251466734));
#14032=CARTESIAN_POINT('Ctrl Pts',(1.31917543061769,1.39539254159618,0.99134926498299));
#14033=CARTESIAN_POINT('Ctrl Pts',(1.30734972067592,1.42347183818157,1.00672880483252));
#14034=CARTESIAN_POINT('Ctrl Pts',(1.29146042158868,1.48505200040818,1.02703269653942));
#14035=CARTESIAN_POINT('Ctrl Pts',(1.28744468918255,1.51855708359447,1.03198167246111));
#14036=CARTESIAN_POINT('Ctrl Pts',(1.28744468918255,1.58144291640553,1.03198167246111));
#14037=CARTESIAN_POINT('Ctrl Pts',(1.29146042158868,1.61494799959182,1.02703269653942));
#14038=CARTESIAN_POINT('Ctrl Pts',(1.30734972067592,1.67652816181843,1.00672880483252));
#14039=CARTESIAN_POINT('Ctrl Pts',(1.31917543061769,1.70460745840382,0.991349264982991));
#14040=CARTESIAN_POINT('Ctrl Pts',(1.34548213209931,1.74894552961493,0.955340251466735));
#14041=CARTESIAN_POINT('Ctrl Pts',(1.36172049302549,1.76817777258318,0.932292094146256));
#14042=CARTESIAN_POINT('Ctrl Pts',(1.39561049050871,1.79370633789704,0.880751161609749));
#14043=CARTESIAN_POINT('Ctrl Pts',(1.4132207435299,1.8,0.85222986989595));
#14044=CARTESIAN_POINT('Ctrl Pts',(1.42894191624432,1.8,0.825000000000001));
#14045=CARTESIAN_POINT('Ctrl Pts',(1.53744468918255,1.55,0.598968970568896));
#14046=CARTESIAN_POINT('Ctrl Pts',(1.53744468918255,1.51855708359447,0.598968970568896));
#14047=CARTESIAN_POINT('Ctrl Pts',(1.53516661651472,1.48505200040818,0.60492118480825));
#14048=CARTESIAN_POINT('Ctrl Pts',(1.52552758004446,1.42347183818157,0.628833667319578));
#14049=CARTESIAN_POINT('Ctrl Pts',(1.51812136280714,1.39539254159618,0.646764802471699));
#14050=CARTESIAN_POINT('Ctrl Pts',(1.50008999307766,1.35105447038507,0.687551581002689));
#14051=CARTESIAN_POINT('Ctrl Pts',(1.48824888379079,1.33182222741682,0.713138492740816));
#14052=CARTESIAN_POINT('Ctrl Pts',(1.46055812562105,1.30629366210296,0.768258557763732));
#14053=CARTESIAN_POINT('Ctrl Pts',(1.44466308895875,1.3,0.797770130104052));
#14054=CARTESIAN_POINT('Ctrl Pts',(1.42894191624432,1.3,0.825000000000001));
#14055=CARTESIAN_POINT('',(0.963525491562421,1.55,0.267616567329818));
#14056=CARTESIAN_POINT('',(0.125,1.55,-0.21650635094611));
#14057=CARTESIAN_POINT('Ctrl Pts',(0.963525491562421,1.55,0.267616567329818));
#14058=CARTESIAN_POINT('Ctrl Pts',(0.963525491562421,1.5815373526696,0.267616567329818));
#14059=CARTESIAN_POINT('Ctrl Pts',(0.961833761492987,1.61508042700263,0.273949373987484));
#14060=CARTESIAN_POINT('Ctrl Pts',(0.954308486908894,1.67663267125761,0.299111603474268));
#14061=CARTESIAN_POINT('Ctrl Pts',(0.948394987258249,1.70465411363682,0.31788699900678));
#14062=CARTESIAN_POINT('Ctrl Pts',(0.933155485613026,1.74889618382539,0.360174810895352));
#14063=CARTESIAN_POINT('Ctrl Pts',(0.92278792026947,1.76811531482682,0.386546956384144));
#14064=CARTESIAN_POINT('Ctrl Pts',(0.897143218189782,1.79367084275751,0.442820664919227));
#14065=CARTESIAN_POINT('Ctrl Pts',(0.881791875377343,1.8,0.472691670144998));
#14066=CARTESIAN_POINT('Ctrl Pts',(0.850258932191534,1.8,0.527308329855003));
#14067=CARTESIAN_POINT('Ctrl Pts',(0.832065554235658,1.79367084275751,0.555538485325664));
#14068=CARTESIAN_POINT('Ctrl Pts',(0.796153444118959,1.76811531482682,0.605884303066698));
#14069=CARTESIAN_POINT('Ctrl Pts',(0.778498278845144,1.74889618382539,0.62804895077401));
#14070=CARTESIAN_POINT('Ctrl Pts',(0.749495710301794,1.70465411363682,0.662390652284073));
#14071=CARTESIAN_POINT('Ctrl Pts',(0.73619249062986,1.67663267125761,0.676899590973058));
#14072=CARTESIAN_POINT('Ctrl Pts',(0.718163997970498,1.61508042700263,0.695997784676728));
#14073=CARTESIAN_POINT('Ctrl Pts',(0.713525491562421,1.5815373526696,0.700629269222037));
#14074=CARTESIAN_POINT('Ctrl Pts',(0.713525491562421,1.5184626473304,0.700629269222037));
#14075=CARTESIAN_POINT('Ctrl Pts',(0.718163997970498,1.48491957299737,0.695997784676728));
#14076=CARTESIAN_POINT('Ctrl Pts',(0.73619249062986,1.42336732874239,0.676899590973058));
#14077=CARTESIAN_POINT('Ctrl Pts',(0.749495710301794,1.39534588636318,0.662390652284073));
#14078=CARTESIAN_POINT('Ctrl Pts',(0.778498278845144,1.35110381617461,0.62804895077401));
#14079=CARTESIAN_POINT('Ctrl Pts',(0.796153444118959,1.33188468517318,0.605884303066698));
#14080=CARTESIAN_POINT('Ctrl Pts',(0.832065554235658,1.30632915724249,0.555538485325664));
#14081=CARTESIAN_POINT('Ctrl Pts',(0.850258932191534,1.3,0.527308329855003));
#14082=CARTESIAN_POINT('Ctrl Pts',(0.881791875377343,1.3,0.472691670144998));
#14083=CARTESIAN_POINT('Ctrl Pts',(0.897143218189782,1.30632915724249,0.442820664919227));
#14084=CARTESIAN_POINT('Ctrl Pts',(0.92278792026947,1.33188468517318,0.386546956384144));
#14085=CARTESIAN_POINT('Ctrl Pts',(0.933155485613026,1.35110381617461,0.360174810895352));
#14086=CARTESIAN_POINT('Ctrl Pts',(0.948394987258249,1.39534588636318,0.31788699900678));
#14087=CARTESIAN_POINT('Ctrl Pts',(0.954308486908894,1.42336732874239,0.299111603474268));
#14088=CARTESIAN_POINT('Ctrl Pts',(0.961833761492987,1.48491957299738,0.273949373987484));
#14089=CARTESIAN_POINT('Ctrl Pts',(0.963525491562421,1.5184626473304,0.267616567329818));
#14090=CARTESIAN_POINT('Ctrl Pts',(0.963525491562421,1.55,0.267616567329818));
#14091=CARTESIAN_POINT('Origin',(0.,1.55,0.));
#14092=CARTESIAN_POINT('',(-0.713525491562421,1.55,-0.700629269222037));
#14093=CARTESIAN_POINT('Ctrl Pts',(-0.713525491562421,1.55,-0.700629269222037));
#14094=CARTESIAN_POINT('Ctrl Pts',(-0.713525491562421,1.5184626473304,-0.700629269222037));
#14095=CARTESIAN_POINT('Ctrl Pts',(-0.718163997970498,1.48491957299737,
-0.695997784676728));
#14096=CARTESIAN_POINT('Ctrl Pts',(-0.73619249062986,1.42336732874239,-0.676899590973058));
#14097=CARTESIAN_POINT('Ctrl Pts',(-0.749495710301794,1.39534588636318,
-0.662390652284073));
#14098=CARTESIAN_POINT('Ctrl Pts',(-0.778498278845144,1.35110381617461,
-0.62804895077401));
#14099=CARTESIAN_POINT('Ctrl Pts',(-0.796153444118959,1.33188468517318,
-0.605884303066698));
#14100=CARTESIAN_POINT('Ctrl Pts',(-0.832065554235658,1.30632915724249,
-0.555538485325664));
#14101=CARTESIAN_POINT('Ctrl Pts',(-0.850258932191534,1.3,-0.527308329855003));
#14102=CARTESIAN_POINT('Ctrl Pts',(-0.881791875377343,1.3,-0.472691670144998));
#14103=CARTESIAN_POINT('Ctrl Pts',(-0.897143218189782,1.30632915724249,
-0.442820664919227));
#14104=CARTESIAN_POINT('Ctrl Pts',(-0.92278792026947,1.33188468517318,-0.386546956384144));
#14105=CARTESIAN_POINT('Ctrl Pts',(-0.933155485613026,1.35110381617461,
-0.360174810895352));
#14106=CARTESIAN_POINT('Ctrl Pts',(-0.948394987258249,1.39534588636318,
-0.31788699900678));
#14107=CARTESIAN_POINT('Ctrl Pts',(-0.954308486908894,1.42336732874239,
-0.299111603474268));
#14108=CARTESIAN_POINT('Ctrl Pts',(-0.961833761492986,1.48491957299737,
-0.273949373987484));
#14109=CARTESIAN_POINT('Ctrl Pts',(-0.963525491562421,1.5184626473304,-0.267616567329818));
#14110=CARTESIAN_POINT('Ctrl Pts',(-0.963525491562421,1.5815373526696,-0.267616567329818));
#14111=CARTESIAN_POINT('Ctrl Pts',(-0.961833761492986,1.61508042700263,
-0.273949373987484));
#14112=CARTESIAN_POINT('Ctrl Pts',(-0.954308486908894,1.67663267125761,
-0.299111603474268));
#14113=CARTESIAN_POINT('Ctrl Pts',(-0.948394987258249,1.70465411363682,
-0.31788699900678));
#14114=CARTESIAN_POINT('Ctrl Pts',(-0.933155485613026,1.74889618382539,
-0.360174810895352));
#14115=CARTESIAN_POINT('Ctrl Pts',(-0.92278792026947,1.76811531482682,-0.386546956384144));
#14116=CARTESIAN_POINT('Ctrl Pts',(-0.897143218189782,1.79367084275751,
-0.442820664919227));
#14117=CARTESIAN_POINT('Ctrl Pts',(-0.881791875377343,1.8,-0.472691670144998));
#14118=CARTESIAN_POINT('Ctrl Pts',(-0.850258932191534,1.8,-0.527308329855003));
#14119=CARTESIAN_POINT('Ctrl Pts',(-0.832065554235658,1.79367084275751,
-0.555538485325664));
#14120=CARTESIAN_POINT('Ctrl Pts',(-0.796153444118959,1.76811531482682,
-0.605884303066698));
#14121=CARTESIAN_POINT('Ctrl Pts',(-0.778498278845144,1.74889618382539,
-0.62804895077401));
#14122=CARTESIAN_POINT('Ctrl Pts',(-0.749495710301794,1.70465411363682,
-0.662390652284073));
#14123=CARTESIAN_POINT('Ctrl Pts',(-0.73619249062986,1.67663267125761,-0.676899590973058));
#14124=CARTESIAN_POINT('Ctrl Pts',(-0.718163997970498,1.61508042700263,
-0.695997784676728));
#14125=CARTESIAN_POINT('Ctrl Pts',(-0.713525491562421,1.5815373526696,-0.700629269222037));
#14126=CARTESIAN_POINT('Ctrl Pts',(-0.713525491562421,1.55,-0.700629269222037));
#14127=CARTESIAN_POINT('',(-1.28744468918255,1.55,-1.03198167246111));
#14128=CARTESIAN_POINT('',(0.125,1.55,-0.21650635094611));
#14129=CARTESIAN_POINT('',(-1.42894191624432,1.3,-0.825000000000001));
#14130=CARTESIAN_POINT('Ctrl Pts',(-1.42894191624432,1.3,-0.825000000000001));
#14131=CARTESIAN_POINT('Ctrl Pts',(-1.4132207435299,1.3,-0.852229869895949));
#14132=CARTESIAN_POINT('Ctrl Pts',(-1.39561049050871,1.30629366210296,-0.880751161609749));
#14133=CARTESIAN_POINT('Ctrl Pts',(-1.36172049302549,1.33182222741682,-0.932292094146256));
#14134=CARTESIAN_POINT('Ctrl Pts',(-1.34548213209931,1.35105447038507,-0.955340251466735));
#14135=CARTESIAN_POINT('Ctrl Pts',(-1.31917543061769,1.39539254159618,-0.991349264982991));
#14136=CARTESIAN_POINT('Ctrl Pts',(-1.30734972067592,1.42347183818157,-1.00672880483252));
#14137=CARTESIAN_POINT('Ctrl Pts',(-1.29146042158868,1.48505200040818,-1.02703269653942));
#14138=CARTESIAN_POINT('Ctrl Pts',(-1.28744468918255,1.51855708359447,-1.03198167246111));
#14139=CARTESIAN_POINT('Ctrl Pts',(-1.28744468918255,1.55,-1.03198167246111));
#14140=CARTESIAN_POINT('',(-1.42894191624432,1.8,-0.825000000000001));
#14141=CARTESIAN_POINT('Ctrl Pts',(-1.42894191624432,1.8,-0.825000000000001));
#14142=CARTESIAN_POINT('Ctrl Pts',(-1.44466308895875,1.8,-0.797770130104052));
#14143=CARTESIAN_POINT('Ctrl Pts',(-1.46055812562105,1.79370633789704,-0.768258557763732));
#14144=CARTESIAN_POINT('Ctrl Pts',(-1.48824888379079,1.76817777258318,-0.713138492740816));
#14145=CARTESIAN_POINT('Ctrl Pts',(-1.50008999307766,1.74894552961493,-0.687551581002689));
#14146=CARTESIAN_POINT('Ctrl Pts',(-1.51812136280714,1.70460745840382,-0.646764802471699));
#14147=CARTESIAN_POINT('Ctrl Pts',(-1.52552758004446,1.67652816181843,-0.628833667319578));
#14148=CARTESIAN_POINT('Ctrl Pts',(-1.53516661651472,1.61494799959182,-0.60492118480825));
#14149=CARTESIAN_POINT('Ctrl Pts',(-1.53744468918255,1.58144291640553,-0.598968970568896));
#14150=CARTESIAN_POINT('Ctrl Pts',(-1.53744468918255,1.51855708359447,-0.598968970568896));
#14151=CARTESIAN_POINT('Ctrl Pts',(-1.53516661651472,1.48505200040818,-0.60492118480825));
#14152=CARTESIAN_POINT('Ctrl Pts',(-1.52552758004446,1.42347183818157,-0.628833667319578));
#14153=CARTESIAN_POINT('Ctrl Pts',(-1.51812136280714,1.39539254159618,-0.646764802471699));
#14154=CARTESIAN_POINT('Ctrl Pts',(-1.50008999307766,1.35105447038507,-0.687551581002689));
#14155=CARTESIAN_POINT('Ctrl Pts',(-1.48824888379079,1.33182222741682,-0.713138492740816));
#14156=CARTESIAN_POINT('Ctrl Pts',(-1.46055812562105,1.30629366210296,-0.768258557763732));
#14157=CARTESIAN_POINT('Ctrl Pts',(-1.44466308895875,1.3,-0.797770130104052));
#14158=CARTESIAN_POINT('Ctrl Pts',(-1.42894191624432,1.3,-0.825000000000001));
#14159=CARTESIAN_POINT('Ctrl Pts',(-1.28744468918255,1.55,-1.03198167246111));
#14160=CARTESIAN_POINT('Ctrl Pts',(-1.28744468918255,1.58144291640553,-1.03198167246111));
#14161=CARTESIAN_POINT('Ctrl Pts',(-1.29146042158868,1.61494799959182,-1.02703269653942));
#14162=CARTESIAN_POINT('Ctrl Pts',(-1.30734972067592,1.67652816181843,-1.00672880483252));
#14163=CARTESIAN_POINT('Ctrl Pts',(-1.31917543061769,1.70460745840382,-0.991349264982991));
#14164=CARTESIAN_POINT('Ctrl Pts',(-1.34548213209931,1.74894552961493,-0.955340251466734));
#14165=CARTESIAN_POINT('Ctrl Pts',(-1.36172049302549,1.76817777258318,-0.932292094146256));
#14166=CARTESIAN_POINT('Ctrl Pts',(-1.39561049050871,1.79370633789704,-0.880751161609749));
#14167=CARTESIAN_POINT('Ctrl Pts',(-1.4132207435299,1.8,-0.852229869895949));
#14168=CARTESIAN_POINT('Ctrl Pts',(-1.42894191624432,1.8,-0.825000000000001));
#14169=CARTESIAN_POINT('Origin',(0.,1.55,0.));
#14170=CARTESIAN_POINT('',(-1.65,0.85,-2.02066721859313E-16));
#14171=CARTESIAN_POINT('Origin',(0.,0.85,0.));
#14172=CARTESIAN_POINT('',(-1.65,2.25,-2.02066721859313E-16));
#14173=CARTESIAN_POINT('',(-1.65,1.55,-2.02066721859313E-16));
#14174=CARTESIAN_POINT('Origin',(0.,2.25,0.));
#14175=CARTESIAN_POINT('',(-1.42894191624432,1.3,0.825));
#14176=CARTESIAN_POINT('',(-1.42894191624432,1.8,0.825));
#14177=CARTESIAN_POINT('Ctrl Pts',(-1.42894191624432,1.3,0.825));
#14178=CARTESIAN_POINT('Ctrl Pts',(-1.44466308895875,1.3,0.797770130104051));
#14179=CARTESIAN_POINT('Ctrl Pts',(-1.46055812562105,1.30629366210296,0.768258557763731));
#14180=CARTESIAN_POINT('Ctrl Pts',(-1.48824888379079,1.33182222741682,0.713138492740815));
#14181=CARTESIAN_POINT('Ctrl Pts',(-1.50008999307766,1.35105447038507,0.687551581002688));
#14182=CARTESIAN_POINT('Ctrl Pts',(-1.51812136280714,1.39539254159618,0.646764802471698));
#14183=CARTESIAN_POINT('Ctrl Pts',(-1.52552758004446,1.42347183818157,0.628833667319577));
#14184=CARTESIAN_POINT('Ctrl Pts',(-1.53516661651472,1.48505200040818,0.604921184808249));
#14185=CARTESIAN_POINT('Ctrl Pts',(-1.53744468918255,1.51855708359447,0.598968970568895));
#14186=CARTESIAN_POINT('Ctrl Pts',(-1.53744468918255,1.58144291640553,0.598968970568895));
#14187=CARTESIAN_POINT('Ctrl Pts',(-1.53516661651472,1.61494799959182,0.604921184808249));
#14188=CARTESIAN_POINT('Ctrl Pts',(-1.52552758004446,1.67652816181843,0.628833667319577));
#14189=CARTESIAN_POINT('Ctrl Pts',(-1.51812136280714,1.70460745840382,0.646764802471698));
#14190=CARTESIAN_POINT('Ctrl Pts',(-1.50008999307766,1.74894552961493,0.687551581002688));
#14191=CARTESIAN_POINT('Ctrl Pts',(-1.48824888379079,1.76817777258318,0.713138492740815));
#14192=CARTESIAN_POINT('Ctrl Pts',(-1.46055812562105,1.79370633789704,0.768258557763731));
#14193=CARTESIAN_POINT('Ctrl Pts',(-1.44466308895875,1.8,0.797770130104051));
#14194=CARTESIAN_POINT('Ctrl Pts',(-1.42894191624432,1.8,0.825));
#14195=CARTESIAN_POINT('',(-1.28744468918255,1.55,1.03198167246111));
#14196=CARTESIAN_POINT('Ctrl Pts',(-1.42894191624432,1.8,0.825));
#14197=CARTESIAN_POINT('Ctrl Pts',(-1.4132207435299,1.8,0.852229869895948));
#14198=CARTESIAN_POINT('Ctrl Pts',(-1.39561049050871,1.79370633789704,0.880751161609747));
#14199=CARTESIAN_POINT('Ctrl Pts',(-1.36172049302549,1.76817777258318,0.932292094146255));
#14200=CARTESIAN_POINT('Ctrl Pts',(-1.34548213209931,1.74894552961493,0.955340251466733));
#14201=CARTESIAN_POINT('Ctrl Pts',(-1.31917543061769,1.70460745840382,0.991349264982989));
#14202=CARTESIAN_POINT('Ctrl Pts',(-1.30734972067592,1.67652816181843,1.00672880483252));
#14203=CARTESIAN_POINT('Ctrl Pts',(-1.29146042158868,1.61494799959182,1.02703269653942));
#14204=CARTESIAN_POINT('Ctrl Pts',(-1.28744468918255,1.58144291640553,1.03198167246111));
#14205=CARTESIAN_POINT('Ctrl Pts',(-1.28744468918255,1.55,1.03198167246111));
#14206=CARTESIAN_POINT('Ctrl Pts',(-1.28744468918255,1.55,1.03198167246111));
#14207=CARTESIAN_POINT('Ctrl Pts',(-1.28744468918255,1.51855708359447,1.03198167246111));
#14208=CARTESIAN_POINT('Ctrl Pts',(-1.29146042158868,1.48505200040818,1.02703269653942));
#14209=CARTESIAN_POINT('Ctrl Pts',(-1.30734972067592,1.42347183818157,1.00672880483252));
#14210=CARTESIAN_POINT('Ctrl Pts',(-1.31917543061769,1.39539254159618,0.99134926498299));
#14211=CARTESIAN_POINT('Ctrl Pts',(-1.34548213209931,1.35105447038508,0.955340251466733));
#14212=CARTESIAN_POINT('Ctrl Pts',(-1.36172049302549,1.33182222741682,0.932292094146255));
#14213=CARTESIAN_POINT('Ctrl Pts',(-1.39561049050871,1.30629366210296,0.880751161609748));
#14214=CARTESIAN_POINT('Ctrl Pts',(-1.4132207435299,1.3,0.852229869895949));
#14215=CARTESIAN_POINT('Ctrl Pts',(-1.42894191624432,1.3,0.825));
#14216=CARTESIAN_POINT('',(1.42894191624432,1.8,-0.825));
#14217=CARTESIAN_POINT('',(1.42894191624432,1.3,-0.825));
#14218=CARTESIAN_POINT('Ctrl Pts',(1.42894191624432,1.8,-0.825));
#14219=CARTESIAN_POINT('Ctrl Pts',(1.4132207435299,1.8,-0.852229869895949));
#14220=CARTESIAN_POINT('Ctrl Pts',(1.39561049050871,1.79370633789704,-0.880751161609748));
#14221=CARTESIAN_POINT('Ctrl Pts',(1.36172049302549,1.76817777258318,-0.932292094146255));
#14222=CARTESIAN_POINT('Ctrl Pts',(1.34548213209931,1.74894552961493,-0.955340251466734));
#14223=CARTESIAN_POINT('Ctrl Pts',(1.31917543061769,1.70460745840382,-0.99134926498299));
#14224=CARTESIAN_POINT('Ctrl Pts',(1.30734972067592,1.67652816181843,-1.00672880483252));
#14225=CARTESIAN_POINT('Ctrl Pts',(1.29146042158868,1.61494799959182,-1.02703269653942));
#14226=CARTESIAN_POINT('Ctrl Pts',(1.28744468918255,1.58144291640553,-1.03198167246111));
#14227=CARTESIAN_POINT('Ctrl Pts',(1.28744468918255,1.51855708359447,-1.03198167246111));
#14228=CARTESIAN_POINT('Ctrl Pts',(1.29146042158868,1.48505200040818,-1.02703269653942));
#14229=CARTESIAN_POINT('Ctrl Pts',(1.30734972067592,1.42347183818157,-1.00672880483252));
#14230=CARTESIAN_POINT('Ctrl Pts',(1.31917543061769,1.39539254159618,-0.99134926498299));
#14231=CARTESIAN_POINT('Ctrl Pts',(1.34548213209931,1.35105447038507,-0.955340251466734));
#14232=CARTESIAN_POINT('Ctrl Pts',(1.36172049302549,1.33182222741682,-0.932292094146255));
#14233=CARTESIAN_POINT('Ctrl Pts',(1.39561049050871,1.30629366210296,-0.880751161609748));
#14234=CARTESIAN_POINT('Ctrl Pts',(1.4132207435299,1.3,-0.852229869895948));
#14235=CARTESIAN_POINT('Ctrl Pts',(1.42894191624432,1.3,-0.825));
#14236=CARTESIAN_POINT('',(1.53744468918255,1.55,-0.598968970568895));
#14237=CARTESIAN_POINT('Ctrl Pts',(1.42894191624432,1.3,-0.825));
#14238=CARTESIAN_POINT('Ctrl Pts',(1.44466308895875,1.3,-0.797770130104051));
#14239=CARTESIAN_POINT('Ctrl Pts',(1.46055812562105,1.30629366210296,-0.768258557763731));
#14240=CARTESIAN_POINT('Ctrl Pts',(1.48824888379079,1.33182222741682,-0.713138492740815));
#14241=CARTESIAN_POINT('Ctrl Pts',(1.50008999307766,1.35105447038507,-0.687551581002688));
#14242=CARTESIAN_POINT('Ctrl Pts',(1.51812136280714,1.39539254159618,-0.646764802471698));
#14243=CARTESIAN_POINT('Ctrl Pts',(1.52552758004446,1.42347183818157,-0.628833667319577));
#14244=CARTESIAN_POINT('Ctrl Pts',(1.53516661651472,1.48505200040818,-0.604921184808249));
#14245=CARTESIAN_POINT('Ctrl Pts',(1.53744468918255,1.51855708359447,-0.598968970568895));
#14246=CARTESIAN_POINT('Ctrl Pts',(1.53744468918255,1.55,-0.598968970568895));
#14247=CARTESIAN_POINT('Ctrl Pts',(1.53744468918255,1.55,-0.598968970568895));
#14248=CARTESIAN_POINT('Ctrl Pts',(1.53744468918255,1.58144291640553,-0.598968970568895));
#14249=CARTESIAN_POINT('Ctrl Pts',(1.53516661651472,1.61494799959182,-0.604921184808249));
#14250=CARTESIAN_POINT('Ctrl Pts',(1.52552758004446,1.67652816181843,-0.628833667319577));
#14251=CARTESIAN_POINT('Ctrl Pts',(1.51812136280714,1.70460745840382,-0.646764802471698));
#14252=CARTESIAN_POINT('Ctrl Pts',(1.50008999307766,1.74894552961493,-0.687551581002688));
#14253=CARTESIAN_POINT('Ctrl Pts',(1.48824888379079,1.76817777258318,-0.713138492740815));
#14254=CARTESIAN_POINT('Ctrl Pts',(1.46055812562105,1.79370633789704,-0.768258557763731));
#14255=CARTESIAN_POINT('Ctrl Pts',(1.44466308895875,1.8,-0.797770130104051));
#14256=CARTESIAN_POINT('Ctrl Pts',(1.42894191624432,1.8,-0.825));
#14257=CARTESIAN_POINT('',(0.,1.3,-1.65));
#14258=CARTESIAN_POINT('',(0.,1.8,-1.65));
#14259=CARTESIAN_POINT('Ctrl Pts',(1.38777878078145E-17,1.3,-1.65));
#14260=CARTESIAN_POINT('Ctrl Pts',(0.0314423454288489,1.3,-1.65));
#14261=CARTESIAN_POINT('Ctrl Pts',(0.0649476351123396,1.30629366210296,
-1.64900971937348));
#14262=CARTESIAN_POINT('Ctrl Pts',(0.126528390765307,1.33182222741682,-1.64543058688707));
#14263=CARTESIAN_POINT('Ctrl Pts',(0.154607860978348,1.35105447038507,-1.64289183246942));
#14264=CARTESIAN_POINT('Ctrl Pts',(0.198945932189457,1.39539254159618,-1.63811406745469));
#14265=CARTESIAN_POINT('Ctrl Pts',(0.218177859368546,1.42347183818157,-1.63556247215209));
#14266=CARTESIAN_POINT('Ctrl Pts',(0.243706194926033,1.48505200040818,-1.63195388134767));
#14267=CARTESIAN_POINT('Ctrl Pts',(0.25,1.51855708359447,-1.63095064303001));
#14268=CARTESIAN_POINT('Ctrl Pts',(0.25,1.58144291640553,-1.63095064303001));
#14269=CARTESIAN_POINT('Ctrl Pts',(0.243706194926033,1.61494799959182,-1.63195388134767));
#14270=CARTESIAN_POINT('Ctrl Pts',(0.218177859368546,1.67652816181843,-1.63556247215209));
#14271=CARTESIAN_POINT('Ctrl Pts',(0.198945932189457,1.70460745840382,-1.63811406745469));
#14272=CARTESIAN_POINT('Ctrl Pts',(0.154607860978349,1.74894552961493,-1.64289183246942));
#14273=CARTESIAN_POINT('Ctrl Pts',(0.126528390765307,1.76817777258318,-1.64543058688707));
#14274=CARTESIAN_POINT('Ctrl Pts',(0.0649476351123398,1.79370633789704,
-1.64900971937348));
#14275=CARTESIAN_POINT('Ctrl Pts',(0.031442345428849,1.8,-1.65));
#14276=CARTESIAN_POINT('Ctrl Pts',(7.63278329429795E-17,1.8,-1.65));
#14277=CARTESIAN_POINT('',(-0.25,1.55,-1.63095064303001));
#14278=CARTESIAN_POINT('Ctrl Pts',(9.0205620750794E-17,1.8,-1.65));
#14279=CARTESIAN_POINT('Ctrl Pts',(-0.0314423454288488,1.8,-1.65));
#14280=CARTESIAN_POINT('Ctrl Pts',(-0.0649476351123396,1.79370633789704,
-1.64900971937348));
#14281=CARTESIAN_POINT('Ctrl Pts',(-0.126528390765307,1.76817777258318,
-1.64543058688707));
#14282=CARTESIAN_POINT('Ctrl Pts',(-0.154607860978348,1.74894552961493,
-1.64289183246942));
#14283=CARTESIAN_POINT('Ctrl Pts',(-0.198945932189456,1.70460745840382,
-1.63811406745469));
#14284=CARTESIAN_POINT('Ctrl Pts',(-0.218177859368546,1.67652816181843,
-1.63556247215209));
#14285=CARTESIAN_POINT('Ctrl Pts',(-0.243706194926033,1.61494799959182,
-1.63195388134767));
#14286=CARTESIAN_POINT('Ctrl Pts',(-0.25,1.58144291640553,-1.63095064303001));
#14287=CARTESIAN_POINT('Ctrl Pts',(-0.25,1.55,-1.63095064303001));
#14288=CARTESIAN_POINT('Ctrl Pts',(-0.25,1.55,-1.63095064303001));
#14289=CARTESIAN_POINT('Ctrl Pts',(-0.25,1.51855708359447,-1.63095064303001));
#14290=CARTESIAN_POINT('Ctrl Pts',(-0.243706194926033,1.48505200040818,
-1.63195388134767));
#14291=CARTESIAN_POINT('Ctrl Pts',(-0.218177859368546,1.42347183818157,
-1.63556247215209));
#14292=CARTESIAN_POINT('Ctrl Pts',(-0.198945932189457,1.39539254159618,
-1.63811406745469));
#14293=CARTESIAN_POINT('Ctrl Pts',(-0.154607860978349,1.35105447038507,
-1.64289183246942));
#14294=CARTESIAN_POINT('Ctrl Pts',(-0.126528390765307,1.33182222741682,
-1.64543058688707));
#14295=CARTESIAN_POINT('Ctrl Pts',(-0.0649476351123398,1.30629366210296,
-1.64900971937348));
#14296=CARTESIAN_POINT('Ctrl Pts',(-0.031442345428849,1.3,-1.65));
#14297=CARTESIAN_POINT('Ctrl Pts',(-4.85722573273506E-17,1.3,-1.65));
#14298=CARTESIAN_POINT('',(0.,1.8,1.65));
#14299=CARTESIAN_POINT('',(0.,1.3,1.65));
#14300=CARTESIAN_POINT('Ctrl Pts',(8.32667268468867E-17,1.8,1.65));
#14301=CARTESIAN_POINT('Ctrl Pts',(0.031442345428849,1.8,1.65));
#14302=CARTESIAN_POINT('Ctrl Pts',(0.0649476351123398,1.79370633789704,
1.64900971937348));
#14303=CARTESIAN_POINT('Ctrl Pts',(0.126528390765307,1.76817777258318,1.64543058688707));
#14304=CARTESIAN_POINT('Ctrl Pts',(0.154607860978349,1.74894552961493,1.64289183246942));
#14305=CARTESIAN_POINT('Ctrl Pts',(0.198945932189457,1.70460745840382,1.63811406745469));
#14306=CARTESIAN_POINT('Ctrl Pts',(0.218177859368546,1.67652816181843,1.63556247215209));
#14307=CARTESIAN_POINT('Ctrl Pts',(0.243706194926033,1.61494799959182,1.63195388134767));
#14308=CARTESIAN_POINT('Ctrl Pts',(0.25,1.58144291640553,1.63095064303001));
#14309=CARTESIAN_POINT('Ctrl Pts',(0.25,1.51855708359447,1.63095064303001));
#14310=CARTESIAN_POINT('Ctrl Pts',(0.243706194926033,1.48505200040818,1.63195388134767));
#14311=CARTESIAN_POINT('Ctrl Pts',(0.218177859368546,1.42347183818157,1.63556247215209));
#14312=CARTESIAN_POINT('Ctrl Pts',(0.198945932189457,1.39539254159618,1.63811406745469));
#14313=CARTESIAN_POINT('Ctrl Pts',(0.154607860978348,1.35105447038507,1.64289183246942));
#14314=CARTESIAN_POINT('Ctrl Pts',(0.126528390765307,1.33182222741682,1.64543058688707));
#14315=CARTESIAN_POINT('Ctrl Pts',(0.0649476351123397,1.30629366210296,
1.64900971937348));
#14316=CARTESIAN_POINT('Ctrl Pts',(0.0314423454288488,1.3,1.65));
#14317=CARTESIAN_POINT('Ctrl Pts',(-1.38777878078145E-17,1.3,1.65));
#14318=CARTESIAN_POINT('',(-0.25,1.55,1.63095064303001));
#14319=CARTESIAN_POINT('Ctrl Pts',(-5.55111512312578E-17,1.3,1.65));
#14320=CARTESIAN_POINT('Ctrl Pts',(-0.031442345428849,1.3,1.65));
#14321=CARTESIAN_POINT('Ctrl Pts',(-0.0649476351123398,1.30629366210296,
1.64900971937348));
#14322=CARTESIAN_POINT('Ctrl Pts',(-0.126528390765307,1.33182222741682,
1.64543058688707));
#14323=CARTESIAN_POINT('Ctrl Pts',(-0.154607860978349,1.35105447038507,
1.64289183246942));
#14324=CARTESIAN_POINT('Ctrl Pts',(-0.198945932189457,1.39539254159618,
1.63811406745469));
#14325=CARTESIAN_POINT('Ctrl Pts',(-0.218177859368546,1.42347183818157,
1.63556247215209));
#14326=CARTESIAN_POINT('Ctrl Pts',(-0.243706194926033,1.48505200040818,
1.63195388134767));
#14327=CARTESIAN_POINT('Ctrl Pts',(-0.25,1.51855708359447,1.63095064303001));
#14328=CARTESIAN_POINT('Ctrl Pts',(-0.25,1.55,1.63095064303001));
#14329=CARTESIAN_POINT('Ctrl Pts',(-0.25,1.55,1.63095064303001));
#14330=CARTESIAN_POINT('Ctrl Pts',(-0.25,1.58144291640553,1.63095064303001));
#14331=CARTESIAN_POINT('Ctrl Pts',(-0.243706194926033,1.61494799959182,
1.63195388134767));
#14332=CARTESIAN_POINT('Ctrl Pts',(-0.218177859368546,1.67652816181843,
1.63556247215209));
#14333=CARTESIAN_POINT('Ctrl Pts',(-0.198945932189456,1.70460745840382,
1.63811406745469));
#14334=CARTESIAN_POINT('Ctrl Pts',(-0.154607860978348,1.74894552961493,
1.64289183246942));
#14335=CARTESIAN_POINT('Ctrl Pts',(-0.126528390765307,1.76817777258318,
1.64543058688707));
#14336=CARTESIAN_POINT('Ctrl Pts',(-0.0649476351123396,1.79370633789704,
1.64900971937348));
#14337=CARTESIAN_POINT('Ctrl Pts',(-0.0314423454288488,1.8,1.65));
#14338=CARTESIAN_POINT('Ctrl Pts',(7.63278329429795E-17,1.8,1.65));
#14339=CARTESIAN_POINT('Origin',(0.,1.55,0.));
#14340=CARTESIAN_POINT('',(-0.713525491562421,1.55,0.700629269222037));
#14341=CARTESIAN_POINT('',(0.125,1.55,0.21650635094611));
#14342=CARTESIAN_POINT('Ctrl Pts',(-0.713525491562421,1.55,0.700629269222037));
#14343=CARTESIAN_POINT('Ctrl Pts',(-0.713525491562421,1.5815373526696,0.700629269222037));
#14344=CARTESIAN_POINT('Ctrl Pts',(-0.718163997970498,1.61508042700263,
0.695997784676727));
#14345=CARTESIAN_POINT('Ctrl Pts',(-0.73619249062986,1.67663267125761,0.676899590973058));
#14346=CARTESIAN_POINT('Ctrl Pts',(-0.749495710301795,1.70465411363682,
0.662390652284073));
#14347=CARTESIAN_POINT('Ctrl Pts',(-0.778498278845144,1.74889618382539,
0.628048950774009));
#14348=CARTESIAN_POINT('Ctrl Pts',(-0.796153444118959,1.76811531482682,
0.605884303066698));
#14349=CARTESIAN_POINT('Ctrl Pts',(-0.832065554235658,1.79367084275751,
0.555538485325663));
#14350=CARTESIAN_POINT('Ctrl Pts',(-0.850258932191534,1.8,0.527308329855002));
#14351=CARTESIAN_POINT('Ctrl Pts',(-0.881791875377343,1.8,0.472691670144998));
#14352=CARTESIAN_POINT('Ctrl Pts',(-0.897143218189782,1.79367084275751,
0.442820664919227));
#14353=CARTESIAN_POINT('Ctrl Pts',(-0.92278792026947,1.76811531482682,0.386546956384144));
#14354=CARTESIAN_POINT('Ctrl Pts',(-0.933155485613026,1.74889618382539,
0.360174810895352));
#14355=CARTESIAN_POINT('Ctrl Pts',(-0.948394987258249,1.70465411363682,
0.31788699900678));
#14356=CARTESIAN_POINT('Ctrl Pts',(-0.954308486908894,1.67663267125761,
0.299111603474267));
#14357=CARTESIAN_POINT('Ctrl Pts',(-0.961833761492987,1.61508042700263,
0.273949373987484));
#14358=CARTESIAN_POINT('Ctrl Pts',(-0.963525491562421,1.5815373526696,0.267616567329817));
#14359=CARTESIAN_POINT('Ctrl Pts',(-0.963525491562421,1.5184626473304,0.267616567329817));
#14360=CARTESIAN_POINT('Ctrl Pts',(-0.961833761492987,1.48491957299737,
0.273949373987484));
#14361=CARTESIAN_POINT('Ctrl Pts',(-0.954308486908894,1.42336732874239,
0.299111603474267));
#14362=CARTESIAN_POINT('Ctrl Pts',(-0.948394987258249,1.39534588636318,
0.31788699900678));
#14363=CARTESIAN_POINT('Ctrl Pts',(-0.933155485613026,1.35110381617461,
0.360174810895352));
#14364=CARTESIAN_POINT('Ctrl Pts',(-0.92278792026947,1.33188468517318,0.386546956384144));
#14365=CARTESIAN_POINT('Ctrl Pts',(-0.897143218189782,1.30632915724249,
0.442820664919227));
#14366=CARTESIAN_POINT('Ctrl Pts',(-0.881791875377343,1.3,0.472691670144998));
#14367=CARTESIAN_POINT('Ctrl Pts',(-0.850258932191534,1.3,0.527308329855002));
#14368=CARTESIAN_POINT('Ctrl Pts',(-0.832065554235658,1.30632915724249,
0.555538485325663));
#14369=CARTESIAN_POINT('Ctrl Pts',(-0.796153444118959,1.33188468517318,
0.605884303066698));
#14370=CARTESIAN_POINT('Ctrl Pts',(-0.778498278845144,1.35110381617461,
0.628048950774009));
#14371=CARTESIAN_POINT('Ctrl Pts',(-0.749495710301795,1.39534588636318,
0.662390652284073));
#14372=CARTESIAN_POINT('Ctrl Pts',(-0.73619249062986,1.42336732874239,0.676899590973058));
#14373=CARTESIAN_POINT('Ctrl Pts',(-0.718163997970498,1.48491957299737,
0.695997784676727));
#14374=CARTESIAN_POINT('Ctrl Pts',(-0.713525491562421,1.5184626473304,0.700629269222037));
#14375=CARTESIAN_POINT('Ctrl Pts',(-0.713525491562421,1.55,0.700629269222037));
#14376=CARTESIAN_POINT('Origin',(0.,1.55,0.));
#14377=CARTESIAN_POINT('',(0.963525491562421,1.55,-0.267616567329817));
#14378=CARTESIAN_POINT('Ctrl Pts',(0.963525491562421,1.55,-0.267616567329817));
#14379=CARTESIAN_POINT('Ctrl Pts',(0.963525491562421,1.5184626473304,-0.267616567329817));
#14380=CARTESIAN_POINT('Ctrl Pts',(0.961833761492987,1.48491957299737,-0.273949373987484));
#14381=CARTESIAN_POINT('Ctrl Pts',(0.954308486908894,1.42336732874239,-0.299111603474267));
#14382=CARTESIAN_POINT('Ctrl Pts',(0.948394987258249,1.39534588636318,-0.31788699900678));
#14383=CARTESIAN_POINT('Ctrl Pts',(0.933155485613026,1.35110381617461,-0.360174810895352));
#14384=CARTESIAN_POINT('Ctrl Pts',(0.92278792026947,1.33188468517318,-0.386546956384144));
#14385=CARTESIAN_POINT('Ctrl Pts',(0.897143218189782,1.30632915724249,-0.442820664919227));
#14386=CARTESIAN_POINT('Ctrl Pts',(0.881791875377343,1.3,-0.472691670144998));
#14387=CARTESIAN_POINT('Ctrl Pts',(0.850258932191534,1.3,-0.527308329855002));
#14388=CARTESIAN_POINT('Ctrl Pts',(0.832065554235658,1.30632915724249,-0.555538485325663));
#14389=CARTESIAN_POINT('Ctrl Pts',(0.796153444118959,1.33188468517318,-0.605884303066698));
#14390=CARTESIAN_POINT('Ctrl Pts',(0.778498278845144,1.35110381617461,-0.628048950774009));
#14391=CARTESIAN_POINT('Ctrl Pts',(0.749495710301795,1.39534588636318,-0.662390652284073));
#14392=CARTESIAN_POINT('Ctrl Pts',(0.73619249062986,1.42336732874239,-0.676899590973058));
#14393=CARTESIAN_POINT('Ctrl Pts',(0.718163997970498,1.48491957299737,-0.695997784676727));
#14394=CARTESIAN_POINT('Ctrl Pts',(0.713525491562421,1.5184626473304,-0.700629269222037));
#14395=CARTESIAN_POINT('Ctrl Pts',(0.713525491562421,1.5815373526696,-0.700629269222037));
#14396=CARTESIAN_POINT('Ctrl Pts',(0.718163997970498,1.61508042700263,-0.695997784676727));
#14397=CARTESIAN_POINT('Ctrl Pts',(0.73619249062986,1.67663267125761,-0.676899590973058));
#14398=CARTESIAN_POINT('Ctrl Pts',(0.749495710301795,1.70465411363682,-0.662390652284073));
#14399=CARTESIAN_POINT('Ctrl Pts',(0.778498278845144,1.74889618382539,-0.628048950774009));
#14400=CARTESIAN_POINT('Ctrl Pts',(0.796153444118959,1.76811531482682,-0.605884303066698));
#14401=CARTESIAN_POINT('Ctrl Pts',(0.832065554235658,1.79367084275751,-0.555538485325663));
#14402=CARTESIAN_POINT('Ctrl Pts',(0.850258932191534,1.8,-0.527308329855002));
#14403=CARTESIAN_POINT('Ctrl Pts',(0.881791875377343,1.8,-0.472691670144998));
#14404=CARTESIAN_POINT('Ctrl Pts',(0.897143218189782,1.79367084275751,-0.442820664919227));
#14405=CARTESIAN_POINT('Ctrl Pts',(0.92278792026947,1.76811531482682,-0.386546956384144));
#14406=CARTESIAN_POINT('Ctrl Pts',(0.933155485613026,1.74889618382539,-0.360174810895352));
#14407=CARTESIAN_POINT('Ctrl Pts',(0.948394987258249,1.70465411363682,-0.31788699900678));
#14408=CARTESIAN_POINT('Ctrl Pts',(0.954308486908894,1.67663267125761,-0.299111603474267));
#14409=CARTESIAN_POINT('Ctrl Pts',(0.961833761492987,1.61508042700263,-0.273949373987484));
#14410=CARTESIAN_POINT('Ctrl Pts',(0.963525491562421,1.5815373526696,-0.267616567329817));
#14411=CARTESIAN_POINT('Ctrl Pts',(0.963525491562421,1.55,-0.267616567329817));
#14412=CARTESIAN_POINT('',(0.125,1.55,0.21650635094611));
#14413=CARTESIAN_POINT('Origin',(0.,1.55,0.));
#14414=CARTESIAN_POINT('',(-0.25,1.55,-0.968245836551854));
#14415=CARTESIAN_POINT('',(-0.25,1.55,0.));
#14416=CARTESIAN_POINT('Ctrl Pts',(-0.25,1.55,-0.968245836551854));
#14417=CARTESIAN_POINT('Ctrl Pts',(-0.25,1.5815373526696,-0.968245836551854));
#14418=CARTESIAN_POINT('Ctrl Pts',(-0.243669763522489,1.61508042700263,
-0.969947158664211));
#14419=CARTESIAN_POINT('Ctrl Pts',(-0.218115996279034,1.67663267125761,
-0.976011194447325));
#14420=CARTESIAN_POINT('Ctrl Pts',(-0.198899276956455,1.70465411363682,
-0.980277651290853));
#14421=CARTESIAN_POINT('Ctrl Pts',(-0.154657206767882,1.74889618382539,
-0.988223761669361));
#14422=CARTESIAN_POINT('Ctrl Pts',(-0.126634476150511,1.76811531482682,
-0.992431259450842));
#14423=CARTESIAN_POINT('Ctrl Pts',(-0.0650776639541238,1.79367084275751,
-0.99835915024489));
#14424=CARTESIAN_POINT('Ctrl Pts',(-0.0315329431858092,1.8,-1.));
#14425=CARTESIAN_POINT('Ctrl Pts',(0.0315329431858092,1.8,-1.));
#14426=CARTESIAN_POINT('Ctrl Pts',(0.0650776639541238,1.79367084275751,
-0.99835915024489));
#14427=CARTESIAN_POINT('Ctrl Pts',(0.126634476150511,1.76811531482682,-0.992431259450842));
#14428=CARTESIAN_POINT('Ctrl Pts',(0.154657206767882,1.74889618382539,-0.988223761669361));
#14429=CARTESIAN_POINT('Ctrl Pts',(0.198899276956455,1.70465411363682,-0.980277651290853));
#14430=CARTESIAN_POINT('Ctrl Pts',(0.218115996279034,1.67663267125761,-0.976011194447325));
#14431=CARTESIAN_POINT('Ctrl Pts',(0.243669763522488,1.61508042700263,-0.969947158664211));
#14432=CARTESIAN_POINT('Ctrl Pts',(0.25,1.5815373526696,-0.968245836551854));
#14433=CARTESIAN_POINT('Ctrl Pts',(0.25,1.5184626473304,-0.968245836551854));
#14434=CARTESIAN_POINT('Ctrl Pts',(0.243669763522488,1.48491957299737,-0.969947158664211));
#14435=CARTESIAN_POINT('Ctrl Pts',(0.218115996279034,1.42336732874239,-0.976011194447325));
#14436=CARTESIAN_POINT('Ctrl Pts',(0.198899276956455,1.39534588636318,-0.980277651290853));
#14437=CARTESIAN_POINT('Ctrl Pts',(0.154657206767882,1.35110381617461,-0.988223761669361));
#14438=CARTESIAN_POINT('Ctrl Pts',(0.126634476150511,1.33188468517318,-0.992431259450842));
#14439=CARTESIAN_POINT('Ctrl Pts',(0.0650776639541239,1.30632915724249,
-0.99835915024489));
#14440=CARTESIAN_POINT('Ctrl Pts',(0.0315329431858092,1.3,-1.));
#14441=CARTESIAN_POINT('Ctrl Pts',(-0.0315329431858092,1.3,-1.));
#14442=CARTESIAN_POINT('Ctrl Pts',(-0.0650776639541239,1.30632915724249,
-0.99835915024489));
#14443=CARTESIAN_POINT('Ctrl Pts',(-0.126634476150511,1.33188468517318,
-0.992431259450842));
#14444=CARTESIAN_POINT('Ctrl Pts',(-0.154657206767882,1.35110381617461,
-0.988223761669361));
#14445=CARTESIAN_POINT('Ctrl Pts',(-0.198899276956455,1.39534588636318,
-0.980277651290853));
#14446=CARTESIAN_POINT('Ctrl Pts',(-0.218115996279034,1.42336732874239,
-0.976011194447325));
#14447=CARTESIAN_POINT('Ctrl Pts',(-0.243669763522489,1.48491957299737,
-0.969947158664211));
#14448=CARTESIAN_POINT('Ctrl Pts',(-0.25,1.5184626473304,-0.968245836551854));
#14449=CARTESIAN_POINT('Ctrl Pts',(-0.25,1.55,-0.968245836551854));
#14450=CARTESIAN_POINT('Origin',(0.,1.55,0.));
#14451=CARTESIAN_POINT('',(-0.25,1.55,0.968245836551854));
#14452=CARTESIAN_POINT('Ctrl Pts',(-0.25,1.55,0.968245836551854));
#14453=CARTESIAN_POINT('Ctrl Pts',(-0.25,1.5184626473304,0.968245836551854));
#14454=CARTESIAN_POINT('Ctrl Pts',(-0.243669763522489,1.48491957299737,
0.969947158664211));
#14455=CARTESIAN_POINT('Ctrl Pts',(-0.218115996279034,1.42336732874239,
0.976011194447325));
#14456=CARTESIAN_POINT('Ctrl Pts',(-0.198899276956455,1.39534588636318,
0.980277651290853));
#14457=CARTESIAN_POINT('Ctrl Pts',(-0.154657206767882,1.35110381617461,
0.988223761669361));
#14458=CARTESIAN_POINT('Ctrl Pts',(-0.126634476150511,1.33188468517318,
0.992431259450842));
#14459=CARTESIAN_POINT('Ctrl Pts',(-0.065077663954124,1.30632915724249,
0.99835915024489));
#14460=CARTESIAN_POINT('Ctrl Pts',(-0.0315329431858092,1.3,1.));
#14461=CARTESIAN_POINT('Ctrl Pts',(0.0315329431858092,1.3,1.));
#14462=CARTESIAN_POINT('Ctrl Pts',(0.065077663954124,1.30632915724249,0.99835915024489));
#14463=CARTESIAN_POINT('Ctrl Pts',(0.126634476150511,1.33188468517318,0.992431259450842));
#14464=CARTESIAN_POINT('Ctrl Pts',(0.154657206767882,1.35110381617461,0.988223761669361));
#14465=CARTESIAN_POINT('Ctrl Pts',(0.198899276956455,1.39534588636318,0.980277651290853));
#14466=CARTESIAN_POINT('Ctrl Pts',(0.218115996279034,1.42336732874239,0.976011194447325));
#14467=CARTESIAN_POINT('Ctrl Pts',(0.243669763522488,1.48491957299737,0.969947158664211));
#14468=CARTESIAN_POINT('Ctrl Pts',(0.25,1.5184626473304,0.968245836551854));
#14469=CARTESIAN_POINT('Ctrl Pts',(0.25,1.5815373526696,0.968245836551854));
#14470=CARTESIAN_POINT('Ctrl Pts',(0.243669763522488,1.61508042700263,0.969947158664211));
#14471=CARTESIAN_POINT('Ctrl Pts',(0.218115996279034,1.67663267125761,0.976011194447325));
#14472=CARTESIAN_POINT('Ctrl Pts',(0.198899276956455,1.70465411363682,0.980277651290853));
#14473=CARTESIAN_POINT('Ctrl Pts',(0.154657206767882,1.74889618382539,0.988223761669361));
#14474=CARTESIAN_POINT('Ctrl Pts',(0.126634476150511,1.76811531482682,0.992431259450842));
#14475=CARTESIAN_POINT('Ctrl Pts',(0.0650776639541239,1.79367084275751,
0.99835915024489));
#14476=CARTESIAN_POINT('Ctrl Pts',(0.0315329431858092,1.8,1.));
#14477=CARTESIAN_POINT('Ctrl Pts',(-0.0315329431858092,1.8,1.));
#14478=CARTESIAN_POINT('Ctrl Pts',(-0.0650776639541239,1.79367084275751,
0.99835915024489));
#14479=CARTESIAN_POINT('Ctrl Pts',(-0.126634476150511,1.76811531482682,
0.992431259450842));
#14480=CARTESIAN_POINT('Ctrl Pts',(-0.154657206767882,1.74889618382539,
0.988223761669361));
#14481=CARTESIAN_POINT('Ctrl Pts',(-0.198899276956455,1.70465411363682,
0.980277651290853));
#14482=CARTESIAN_POINT('Ctrl Pts',(-0.218115996279034,1.67663267125761,
0.976011194447325));
#14483=CARTESIAN_POINT('Ctrl Pts',(-0.243669763522489,1.61508042700263,
0.969947158664211));
#14484=CARTESIAN_POINT('Ctrl Pts',(-0.25,1.5815373526696,0.968245836551854));
#14485=CARTESIAN_POINT('Ctrl Pts',(-0.25,1.55,0.968245836551854));
#14486=CARTESIAN_POINT('',(-0.25,1.55,0.));
#14487=CARTESIAN_POINT('Origin',(1.65,2.25,0.));
#14488=CARTESIAN_POINT('',(-1.,2.25,-1.22464679914735E-16));
#14489=CARTESIAN_POINT('Origin',(0.,2.25,0.));
#14490=CARTESIAN_POINT('Origin',(1.75,0.85,0.));
#14491=CARTESIAN_POINT('',(-1.75,0.85,-2.14313189850787E-16));
#14492=CARTESIAN_POINT('Origin',(0.,0.85,0.));
#14493=CARTESIAN_POINT('Origin',(0.,0.,0.));
#14494=CARTESIAN_POINT('',(-1.75,-0.85,-2.14313189850787E-16));
#14495=CARTESIAN_POINT('Origin',(0.,-0.85,0.));
#14496=CARTESIAN_POINT('',(-1.75,0.,-2.14313189850787E-16));
#14497=CARTESIAN_POINT('Origin',(1.,-0.85,0.));
#14498=CARTESIAN_POINT('',(-1.,-0.85,-1.22464679914735E-16));
#14499=CARTESIAN_POINT('Origin',(0.,-0.85,0.));
#14500=CARTESIAN_POINT('Origin',(0.,0.7,0.));
#14501=CARTESIAN_POINT('',(-1.,0.7,-1.22464679914735E-16));
#16808=UNCERTAINTY_MEASURE_WITH_UNIT(LENGTH_MEASURE(0.001),#16912,
'DISTANCE_ACCURACY_VALUE',
'Maximum model space distance between geometric entities at asserted c
onnectivities');
#16852=UNCERTAINTY_MEASURE_WITH_UNIT(LENGTH_MEASURE(0.001),#16912,
'DISTANCE_ACCURACY_VALUE',
'Maximum model space distance between geometric entities at asserted c
onnectivities');
#16867=(
GEOMETRIC_REPRESENTATION_CONTEXT(3)
GLOBAL_UNCERTAINTY_ASSIGNED_CONTEXT((#16808))
GLOBAL_UNIT_ASSIGNED_CONTEXT((#16912,#16914,#16915))
REPRESENTATION_CONTEXT('','3D')
);
#16911=(
GEOMETRIC_REPRESENTATION_CONTEXT(3)
GLOBAL_UNCERTAINTY_ASSIGNED_CONTEXT((#16852))
GLOBAL_UNIT_ASSIGNED_CONTEXT((#16912,#16914,#16915))
REPRESENTATION_CONTEXT('','3D')
);
#16912=(
LENGTH_UNIT()
NAMED_UNIT(*)
SI_UNIT(.CENTI.,.METRE.)
);
#16914=(
NAMED_UNIT(*)
PLANE_ANGLE_UNIT()
SI_UNIT($,.RADIAN.)
);
#16915=(
NAMED_UNIT(*)
SI_UNIT($,.STERADIAN.)
SOLID_ANGLE_UNIT()
);
#16930=SHAPE_DEFINITION_REPRESENTATION(#16988,#17138);
#16988=PRODUCT_DEFINITION_SHAPE('',$,#17197);
#17138=SHAPE_REPRESENTATION('',(#9767),#16867);
#17182=PRODUCT_DEFINITION_CONTEXT('part definition',#17358,'design');
#17197=PRODUCT_DEFINITION('Insert bearing','Insert bearing',#17255,#17182);
#17255=PRODUCT_DEFINITION_FORMATION('',$,#17374);
#17358=APPLICATION_CONTEXT(
'Core Data for Automotive Mechanical Design Process');
#17359=PRODUCT_CONTEXT('part definition',#17358,'mechanical');
#17374=PRODUCT('Insert bearing','Insert bearing','Insert bearing',(#17359));
#17481=COLOUR_RGB('Grey',0.48,0.52,0.57);
#17482=FILL_AREA_STYLE_COLOUR('',#17481);
#17483=FILL_AREA_STYLE('',(#17482));
#17484=SURFACE_STYLE_FILL_AREA(#17483);
#17485=SURFACE_SIDE_STYLE('',(#17484));
#17486=SURFACE_STYLE_USAGE(.BOTH.,#17485);
#17487=PRESENTATION_STYLE_ASSIGNMENT((#17486));
ENDSEC;
END-ISO-10303-21;
